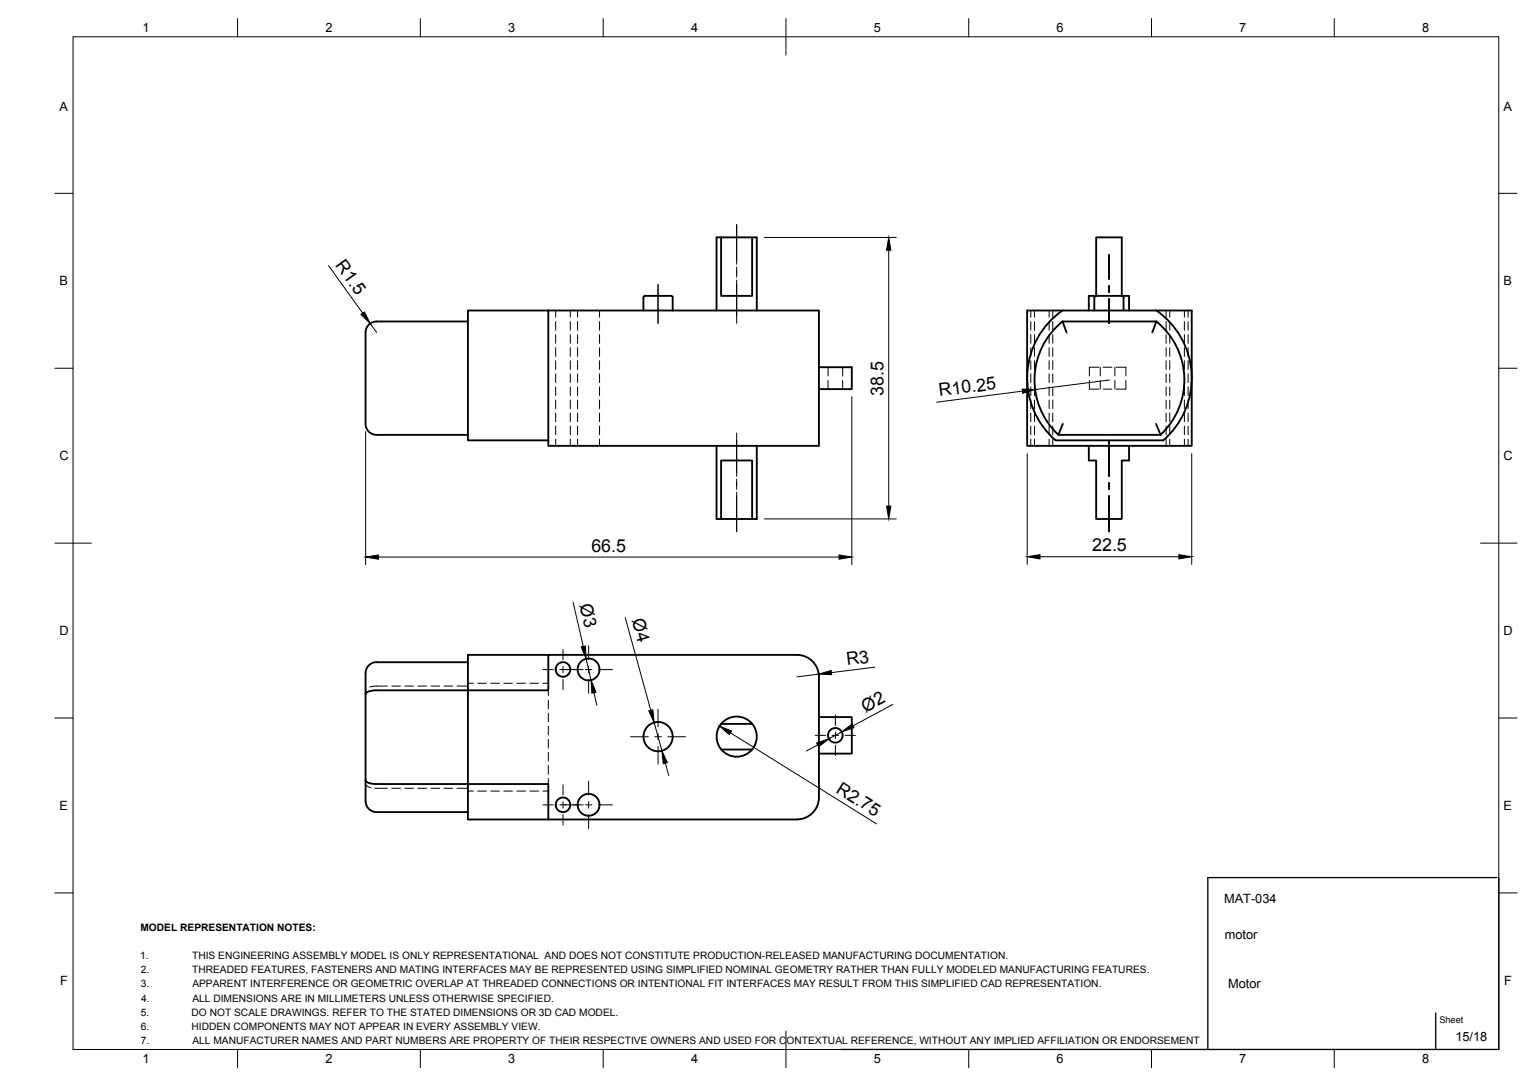
ISO-10303-21;
HEADER;
/* Generated by software containing ST-Developer
 * from STEP Tools, Inc. (www.steptools.com) 
 */

FILE_DESCRIPTION(
/* description */ ('STEP AP214'),
/* implementation_level */ '2;1');

FILE_NAME(
/* name */ 'Motor.step',
/* time_stamp */ '2026-11-14T09:24:36-08:00',
/* author */ (''),
/* organization */ (''),
/* preprocessor_version */ 'ST-DEVELOPER v20.2',
/* originating_system */ 'Autodesk Translation Framework v15.17.0.0',
/* authorisation */ '');

FILE_SCHEMA (('AUTOMOTIVE_DESIGN { 1 0 10303 214 3 1 1 }'));
ENDSEC;

DATA;
#10=MECHANICAL_DESIGN_GEOMETRIC_PRESENTATION_REPRESENTATION('',(#210),#18867);
#142=B_SPLINE_CURVE_WITH_KNOTS('',3,(#16841,#16842,#16843,#16844,#16845,
#16846,#16847,#16848,#16849,#16850,#16851,#16852,#16853,#16854),
 .UNSPECIFIED.,.F.,.F.,(4,2,2,2,2,2,4),(0.245799129465821,0.300704982929502,
0.357513955396153,0.418543136612542,0.45489286030411,0.491598258931638,
0.492200531214483),.UNSPECIFIED.);
#143=B_SPLINE_CURVE_WITH_KNOTS('',3,(#16857,#16858,#16859,#16860,#16861,
#16862,#16863,#16864,#16865,#16866,#16867,#16868,#16869,#16870),
 .UNSPECIFIED.,.F.,.F.,(4,2,2,2,2,2,4),(-0.243764588636152,-0.188160877929009,
-0.130985417478992,-0.0703706382818566,-0.0353193180725583,0.,0.000595335954832901),
 .UNSPECIFIED.);
#144=B_SPLINE_CURVE_WITH_KNOTS('',3,(#17002,#17003,#17004,#17005,#17006,
#17007,#17008,#17009,#17010,#17011,#17012,#17013,#17014,#17015),
 .UNSPECIFIED.,.F.,.F.,(4,2,2,2,2,2,4),(-0.000602272282836634,0.,0.0367053986270638,
0.0730551223181225,0.134084303533662,0.190893275999521,0.245799129462431),
 .UNSPECIFIED.);
#145=B_SPLINE_CURVE_WITH_KNOTS('',3,(#17017,#17018,#17019,#17020,#17021,
#17022,#17023,#17024,#17025,#17026,#17027,#17028,#17029,#17030),
 .UNSPECIFIED.,.F.,.F.,(4,2,2,2,2,2,4),(-0.488124513225642,-0.487529177270534,
-0.452209859198347,-0.417158538989302,-0.356543759792373,-0.299368299342555,
-0.243764588635598),.UNSPECIFIED.);
#154=TOROIDAL_SURFACE('',#11579,1.8,0.2);
#155=TOROIDAL_SURFACE('',#11608,8.75000000000038,1.5);
#156=TOROIDAL_SURFACE('',#11653,8.75000000000038,1.5);
#178=SHAPE_REPRESENTATION_RELATIONSHIP('SRR','None',#18942,#194);
#194=ADVANCED_BREP_SHAPE_REPRESENTATION('',(#234),#18858);
#210=STYLED_ITEM('',(#19026),#234);
#234=MANIFOLD_SOLID_BREP('Body1',#10965);
#327=FACE_BOUND('',#1639,.T.);
#328=FACE_BOUND('',#1640,.T.);
#329=FACE_BOUND('',#1641,.T.);
#330=FACE_BOUND('',#1642,.T.);
#331=FACE_BOUND('',#1643,.T.);
#332=FACE_BOUND('',#1644,.T.);
#333=FACE_BOUND('',#1646,.T.);
#334=FACE_BOUND('',#1649,.T.);
#335=FACE_BOUND('',#1659,.T.);
#336=FACE_BOUND('',#1660,.T.);
#337=FACE_BOUND('',#1661,.T.);
#338=FACE_BOUND('',#1662,.T.);
#339=FACE_BOUND('',#1663,.T.);
#340=FACE_BOUND('',#1682,.T.);
#341=FACE_BOUND('',#1685,.T.);
#523=PLANE('',#11625);
#524=PLANE('',#11628);
#525=PLANE('',#11629);
#526=PLANE('',#11630);
#527=PLANE('',#11636);
#528=PLANE('',#11637);
#529=PLANE('',#11638);
#530=PLANE('',#11639);
#531=PLANE('',#11644);
#532=PLANE('',#11645);
#533=PLANE('',#11646);
#534=PLANE('',#11648);
#535=PLANE('',#11649);
#536=PLANE('',#11650);
#537=PLANE('',#11655);
#538=PLANE('',#11656);
#539=PLANE('',#11657);
#540=PLANE('',#11658);
#541=PLANE('',#11659);
#542=PLANE('',#11660);
#543=PLANE('',#11661);
#544=PLANE('',#11662);
#545=PLANE('',#11663);
#546=PLANE('',#11664);
#547=PLANE('',#11665);
#548=PLANE('',#11666);
#549=PLANE('',#11667);
#550=PLANE('',#11668);
#551=PLANE('',#11669);
#954=FACE_OUTER_BOUND('',#1626,.T.);
#955=FACE_OUTER_BOUND('',#1627,.T.);
#956=FACE_OUTER_BOUND('',#1628,.T.);
#957=FACE_OUTER_BOUND('',#1629,.T.);
#958=FACE_OUTER_BOUND('',#1630,.T.);
#959=FACE_OUTER_BOUND('',#1631,.T.);
#960=FACE_OUTER_BOUND('',#1632,.T.);
#961=FACE_OUTER_BOUND('',#1633,.T.);
#962=FACE_OUTER_BOUND('',#1634,.T.);
#963=FACE_OUTER_BOUND('',#1635,.T.);
#964=FACE_OUTER_BOUND('',#1636,.T.);
#965=FACE_OUTER_BOUND('',#1637,.T.);
#966=FACE_OUTER_BOUND('',#1638,.T.);
#967=FACE_OUTER_BOUND('',#1645,.T.);
#968=FACE_OUTER_BOUND('',#1647,.T.);
#969=FACE_OUTER_BOUND('',#1648,.T.);
#970=FACE_OUTER_BOUND('',#1650,.T.);
#971=FACE_OUTER_BOUND('',#1651,.T.);
#972=FACE_OUTER_BOUND('',#1652,.T.);
#973=FACE_OUTER_BOUND('',#1653,.T.);
#974=FACE_OUTER_BOUND('',#1654,.T.);
#975=FACE_OUTER_BOUND('',#1655,.T.);
#976=FACE_OUTER_BOUND('',#1656,.T.);
#977=FACE_OUTER_BOUND('',#1657,.T.);
#978=FACE_OUTER_BOUND('',#1658,.T.);
#979=FACE_OUTER_BOUND('',#1664,.T.);
#980=FACE_OUTER_BOUND('',#1665,.T.);
#981=FACE_OUTER_BOUND('',#1666,.T.);
#982=FACE_OUTER_BOUND('',#1667,.T.);
#983=FACE_OUTER_BOUND('',#1668,.T.);
#984=FACE_OUTER_BOUND('',#1669,.T.);
#985=FACE_OUTER_BOUND('',#1670,.T.);
#986=FACE_OUTER_BOUND('',#1671,.T.);
#987=FACE_OUTER_BOUND('',#1672,.T.);
#988=FACE_OUTER_BOUND('',#1673,.T.);
#989=FACE_OUTER_BOUND('',#1674,.T.);
#990=FACE_OUTER_BOUND('',#1675,.T.);
#991=FACE_OUTER_BOUND('',#1676,.T.);
#992=FACE_OUTER_BOUND('',#1677,.T.);
#993=FACE_OUTER_BOUND('',#1678,.T.);
#994=FACE_OUTER_BOUND('',#1679,.T.);
#995=FACE_OUTER_BOUND('',#1680,.T.);
#996=FACE_OUTER_BOUND('',#1681,.T.);
#997=FACE_OUTER_BOUND('',#1683,.T.);
#998=FACE_OUTER_BOUND('',#1684,.T.);
#999=FACE_OUTER_BOUND('',#1686,.T.);
#1000=FACE_OUTER_BOUND('',#1687,.T.);
#1001=FACE_OUTER_BOUND('',#1688,.T.);
#1626=EDGE_LOOP('',(#8226,#8227,#8228,#8229,#8230));
#1627=EDGE_LOOP('',(#8231,#8232,#8233,#8234,#8235));
#1628=EDGE_LOOP('',(#8236,#8237,#8238,#8239));
#1629=EDGE_LOOP('',(#8240,#8241,#8242,#8243));
#1630=EDGE_LOOP('',(#8244,#8245,#8246,#8247));
#1631=EDGE_LOOP('',(#8248,#8249,#8250,#8251));
#1632=EDGE_LOOP('',(#8252,#8253,#8254,#8255));
#1633=EDGE_LOOP('',(#8256,#8257,#8258,#8259,#8260,#8261,#8262,#8263,#8264,
#8265,#8266,#8267));
#1634=EDGE_LOOP('',(#8268,#8269,#8270,#8271));
#1635=EDGE_LOOP('',(#8272,#8273,#8274,#8275));
#1636=EDGE_LOOP('',(#8276,#8277,#8278,#8279,#8280));
#1637=EDGE_LOOP('',(#8281,#8282,#8283,#8284,#8285,#8286,#8287,#8288,#8289,
#8290,#8291,#8292));
#1638=EDGE_LOOP('',(#8293,#8294,#8295,#8296,#8297,#8298,#8299,#8300,#8301,
#8302));
#1639=EDGE_LOOP('',(#8303));
#1640=EDGE_LOOP('',(#8304));
#1641=EDGE_LOOP('',(#8305));
#1642=EDGE_LOOP('',(#8306));
#1643=EDGE_LOOP('',(#8307));
#1644=EDGE_LOOP('',(#8308));
#1645=EDGE_LOOP('',(#8309,#8310,#8311,#8312));
#1646=EDGE_LOOP('',(#8313,#8314,#8315,#8316));
#1647=EDGE_LOOP('',(#8317,#8318,#8319,#8320,#8321));
#1648=EDGE_LOOP('',(#8322,#8323,#8324,#8325));
#1649=EDGE_LOOP('',(#8326,#8327,#8328,#8329));
#1650=EDGE_LOOP('',(#8330,#8331,#8332,#8333,#8334));
#1651=EDGE_LOOP('',(#8335,#8336,#8337));
#1652=EDGE_LOOP('',(#8338,#8339,#8340,#8341,#8342,#8343));
#1653=EDGE_LOOP('',(#8344,#8345,#8346));
#1654=EDGE_LOOP('',(#8347,#8348,#8349,#8350,#8351));
#1655=EDGE_LOOP('',(#8352,#8353,#8354,#8355));
#1656=EDGE_LOOP('',(#8356,#8357,#8358,#8359));
#1657=EDGE_LOOP('',(#8360,#8361,#8362,#8363,#8364));
#1658=EDGE_LOOP('',(#8365,#8366,#8367,#8368,#8369,#8370));
#1659=EDGE_LOOP('',(#8371));
#1660=EDGE_LOOP('',(#8372));
#1661=EDGE_LOOP('',(#8373));
#1662=EDGE_LOOP('',(#8374));
#1663=EDGE_LOOP('',(#8375));
#1664=EDGE_LOOP('',(#8376,#8377,#8378,#8379));
#1665=EDGE_LOOP('',(#8380,#8381,#8382,#8383));
#1666=EDGE_LOOP('',(#8384,#8385,#8386,#8387));
#1667=EDGE_LOOP('',(#8388,#8389,#8390,#8391));
#1668=EDGE_LOOP('',(#8392,#8393,#8394,#8395));
#1669=EDGE_LOOP('',(#8396,#8397,#8398,#8399));
#1670=EDGE_LOOP('',(#8400,#8401,#8402,#8403));
#1671=EDGE_LOOP('',(#8404,#8405,#8406,#8407));
#1672=EDGE_LOOP('',(#8408,#8409,#8410,#8411,#8412));
#1673=EDGE_LOOP('',(#8413,#8414));
#1674=EDGE_LOOP('',(#8415,#8416,#8417,#8418));
#1675=EDGE_LOOP('',(#8419,#8420));
#1676=EDGE_LOOP('',(#8421,#8422,#8423,#8424));
#1677=EDGE_LOOP('',(#8425,#8426,#8427,#8428));
#1678=EDGE_LOOP('',(#8429,#8430));
#1679=EDGE_LOOP('',(#8431,#8432,#8433,#8434));
#1680=EDGE_LOOP('',(#8435,#8436));
#1681=EDGE_LOOP('',(#8437,#8438,#8439,#8440));
#1682=EDGE_LOOP('',(#8441));
#1683=EDGE_LOOP('',(#8442,#8443,#8444,#8445));
#1684=EDGE_LOOP('',(#8446,#8447,#8448,#8449));
#1685=EDGE_LOOP('',(#8450));
#1686=EDGE_LOOP('',(#8451,#8452,#8453,#8454));
#1687=EDGE_LOOP('',(#8455,#8456,#8457,#8458));
#1688=EDGE_LOOP('',(#8459));
#2424=LINE('',#16783,#3438);
#2425=LINE('',#16788,#3439);
#2426=LINE('',#16794,#3440);
#2427=LINE('',#16800,#3441);
#2428=LINE('',#16806,#3442);
#2429=LINE('',#16812,#3443);
#2430=LINE('',#16818,#3444);
#2431=LINE('',#16822,#3445);
#2432=LINE('',#16826,#3446);
#2433=LINE('',#16830,#3447);
#2434=LINE('',#16834,#3448);
#2435=LINE('',#16876,#3449);
#2436=LINE('',#16879,#3450);
#2437=LINE('',#16885,#3451);
#2438=LINE('',#16890,#3452);
#2439=LINE('',#16895,#3453);
#2440=LINE('',#16899,#3454);
#2441=LINE('',#16903,#3455);
#2442=LINE('',#16907,#3456);
#2443=LINE('',#16911,#3457);
#2444=LINE('',#16915,#3458);
#2445=LINE('',#16917,#3459);
#2446=LINE('',#16921,#3460);
#2447=LINE('',#16925,#3461);
#2448=LINE('',#16927,#3462);
#2449=LINE('',#16929,#3463);
#2450=LINE('',#16930,#3464);
#2451=LINE('',#16934,#3465);
#2452=LINE('',#16935,#3466);
#2453=LINE('',#16936,#3467);
#2454=LINE('',#16939,#3468);
#2455=LINE('',#16941,#3469);
#2456=LINE('',#16943,#3470);
#2457=LINE('',#16944,#3471);
#2458=LINE('',#16946,#3472);
#2459=LINE('',#16947,#3473);
#2460=LINE('',#16951,#3474);
#2461=LINE('',#16953,#3475);
#2462=LINE('',#16956,#3476);
#2463=LINE('',#16962,#3477);
#2464=LINE('',#16964,#3478);
#2465=LINE('',#16967,#3479);
#2466=LINE('',#16969,#3480);
#2467=LINE('',#16970,#3481);
#2468=LINE('',#16971,#3482);
#2469=LINE('',#16973,#3483);
#2470=LINE('',#16976,#3484);
#2471=LINE('',#16977,#3485);
#2472=LINE('',#16983,#3486);
#2473=LINE('',#16985,#3487);
#2474=LINE('',#16989,#3488);
#2475=LINE('',#16990,#3489);
#2476=LINE('',#16992,#3490);
#2477=LINE('',#16994,#3491);
#2478=LINE('',#16999,#3492);
#2479=LINE('',#17000,#3493);
#2480=LINE('',#17033,#3494);
#2481=LINE('',#17034,#3495);
#2482=LINE('',#17036,#3496);
#2483=LINE('',#17039,#3497);
#2484=LINE('',#17042,#3498);
#2485=LINE('',#17045,#3499);
#2486=LINE('',#17049,#3500);
#2487=LINE('',#17051,#3501);
#2488=LINE('',#17052,#3502);
#2489=LINE('',#17055,#3503);
#2490=LINE('',#17056,#3504);
#2491=LINE('',#17059,#3505);
#2492=LINE('',#17060,#3506);
#2493=LINE('',#17062,#3507);
#3438=VECTOR('',#13534,2.);
#3439=VECTOR('',#13539,1.);
#3440=VECTOR('',#13546,1.);
#3441=VECTOR('',#13553,1.5);
#3442=VECTOR('',#13560,1.5);
#3443=VECTOR('',#13567,1.);
#3444=VECTOR('',#13574,2.75);
#3445=VECTOR('',#13577,1000.);
#3446=VECTOR('',#13580,1000.);
#3447=VECTOR('',#13583,1000.);
#3448=VECTOR('',#13586,1000.);
#3449=VECTOR('',#13599,1000.);
#3450=VECTOR('',#13602,1000.);
#3451=VECTOR('',#13607,1000.);
#3452=VECTOR('',#13612,1000.);
#3453=VECTOR('',#13617,2.75);
#3454=VECTOR('',#13620,1000.);
#3455=VECTOR('',#13623,1000.);
#3456=VECTOR('',#13626,1000.);
#3457=VECTOR('',#13629,1000.);
#3458=VECTOR('',#13634,1000.);
#3459=VECTOR('',#13635,1000.);
#3460=VECTOR('',#13638,1000.);
#3461=VECTOR('',#13641,1000.);
#3462=VECTOR('',#13642,1000.);
#3463=VECTOR('',#13643,1000.);
#3464=VECTOR('',#13644,1000.);
#3465=VECTOR('',#13647,1000.);
#3466=VECTOR('',#13648,1000.);
#3467=VECTOR('',#13649,1000.);
#3468=VECTOR('',#13650,1000.);
#3469=VECTOR('',#13651,1000.);
#3470=VECTOR('',#13652,1000.);
#3471=VECTOR('',#13653,1000.);
#3472=VECTOR('',#13656,1000.);
#3473=VECTOR('',#13657,1000.);
#3474=VECTOR('',#13662,1000.);
#3475=VECTOR('',#13663,1000.);
#3476=VECTOR('',#13666,1000.);
#3477=VECTOR('',#13673,1000.);
#3478=VECTOR('',#13676,1000.);
#3479=VECTOR('',#13679,1000.);
#3480=VECTOR('',#13680,1000.);
#3481=VECTOR('',#13681,1000.);
#3482=VECTOR('',#13682,1000.);
#3483=VECTOR('',#13685,1000.);
#3484=VECTOR('',#13688,1000.);
#3485=VECTOR('',#13689,1000.);
#3486=VECTOR('',#13698,1000.);
#3487=VECTOR('',#13701,1000.);
#3488=VECTOR('',#13708,1000.);
#3489=VECTOR('',#13709,1000.);
#3490=VECTOR('',#13712,1000.);
#3491=VECTOR('',#13715,1000.);
#3492=VECTOR('',#13720,1000.);
#3493=VECTOR('',#13721,1000.);
#3494=VECTOR('',#13730,1000.);
#3495=VECTOR('',#13731,1000.);
#3496=VECTOR('',#13734,1000.);
#3497=VECTOR('',#13739,1000.);
#3498=VECTOR('',#13744,1000.);
#3499=VECTOR('',#13749,1000.);
#3500=VECTOR('',#13754,1000.);
#3501=VECTOR('',#13755,1000.);
#3502=VECTOR('',#13756,1000.);
#3503=VECTOR('',#13759,1000.);
#3504=VECTOR('',#13760,1000.);
#3505=VECTOR('',#13763,1000.);
#3506=VECTOR('',#13764,1000.);
#3507=VECTOR('',#13767,1000.);
#4253=CIRCLE('',#11580,1.8);
#4254=CIRCLE('',#11581,0.2);
#4255=CIRCLE('',#11582,2.);
#4256=CIRCLE('',#11583,2.);
#4257=CIRCLE('',#11585,2.);
#4258=CIRCLE('',#11587,1.);
#4259=CIRCLE('',#11588,1.);
#4260=CIRCLE('',#11590,1.);
#4261=CIRCLE('',#11591,1.);
#4262=CIRCLE('',#11593,1.5);
#4263=CIRCLE('',#11594,1.5);
#4264=CIRCLE('',#11596,1.5);
#4265=CIRCLE('',#11597,1.5);
#4266=CIRCLE('',#11599,1.);
#4267=CIRCLE('',#11600,1.);
#4268=CIRCLE('',#11602,2.75);
#4269=CIRCLE('',#11603,2.75);
#4270=CIRCLE('',#11604,2.75);
#4271=CIRCLE('',#11605,2.75);
#4272=CIRCLE('',#11606,2.75);
#4273=CIRCLE('',#11607,2.75);
#4274=CIRCLE('',#11609,10.2500000000004);
#4275=CIRCLE('',#11610,8.75000000000038);
#4276=CIRCLE('',#11612,10.2500000000004);
#4277=CIRCLE('',#11613,10.2500000000004);
#4278=CIRCLE('',#11615,11.25);
#4279=CIRCLE('',#11616,11.25);
#4280=CIRCLE('',#11617,11.25);
#4281=CIRCLE('',#11619,2.75);
#4282=CIRCLE('',#11620,2.75);
#4283=CIRCLE('',#11621,2.75);
#4284=CIRCLE('',#11622,2.75);
#4285=CIRCLE('',#11623,2.75);
#4286=CIRCLE('',#11624,2.75);
#4287=CIRCLE('',#11626,3.);
#4288=CIRCLE('',#11627,3.);
#4289=CIRCLE('',#11631,11.25);
#4290=CIRCLE('',#11632,10.2500000000004);
#4291=CIRCLE('',#11634,11.25);
#4292=CIRCLE('',#11635,11.25);
#4293=CIRCLE('',#11641,3.);
#4294=CIRCLE('',#11643,3.);
#4295=CIRCLE('',#11651,8.75000000000038);
#4944=VERTEX_POINT('',#16773);
#4945=VERTEX_POINT('',#16775);
#4946=VERTEX_POINT('',#16777);
#4947=VERTEX_POINT('',#16781);
#4948=VERTEX_POINT('',#16785);
#4949=VERTEX_POINT('',#16787);
#4950=VERTEX_POINT('',#16791);
#4951=VERTEX_POINT('',#16793);
#4952=VERTEX_POINT('',#16797);
#4953=VERTEX_POINT('',#16799);
#4954=VERTEX_POINT('',#16803);
#4955=VERTEX_POINT('',#16805);
#4956=VERTEX_POINT('',#16809);
#4957=VERTEX_POINT('',#16811);
#4958=VERTEX_POINT('',#16815);
#4959=VERTEX_POINT('',#16817);
#4960=VERTEX_POINT('',#16819);
#4961=VERTEX_POINT('',#16821);
#4962=VERTEX_POINT('',#16823);
#4963=VERTEX_POINT('',#16825);
#4964=VERTEX_POINT('',#16827);
#4965=VERTEX_POINT('',#16829);
#4966=VERTEX_POINT('',#16831);
#4967=VERTEX_POINT('',#16833);
#4968=VERTEX_POINT('',#16837);
#4969=VERTEX_POINT('',#16838);
#4970=VERTEX_POINT('',#16840);
#4971=VERTEX_POINT('',#16855);
#4972=VERTEX_POINT('',#16872);
#4973=VERTEX_POINT('',#16873);
#4974=VERTEX_POINT('',#16875);
#4975=VERTEX_POINT('',#16877);
#4976=VERTEX_POINT('',#16881);
#4977=VERTEX_POINT('',#16882);
#4978=VERTEX_POINT('',#16884);
#4979=VERTEX_POINT('',#16886);
#4980=VERTEX_POINT('',#16888);
#4981=VERTEX_POINT('',#16892);
#4982=VERTEX_POINT('',#16894);
#4983=VERTEX_POINT('',#16896);
#4984=VERTEX_POINT('',#16898);
#4985=VERTEX_POINT('',#16900);
#4986=VERTEX_POINT('',#16902);
#4987=VERTEX_POINT('',#16904);
#4988=VERTEX_POINT('',#16906);
#4989=VERTEX_POINT('',#16908);
#4990=VERTEX_POINT('',#16910);
#4991=VERTEX_POINT('',#16914);
#4992=VERTEX_POINT('',#16916);
#4993=VERTEX_POINT('',#16918);
#4994=VERTEX_POINT('',#16920);
#4995=VERTEX_POINT('',#16922);
#4996=VERTEX_POINT('',#16924);
#4997=VERTEX_POINT('',#16926);
#4998=VERTEX_POINT('',#16928);
#4999=VERTEX_POINT('',#16932);
#5000=VERTEX_POINT('',#16933);
#5001=VERTEX_POINT('',#16937);
#5002=VERTEX_POINT('',#16938);
#5003=VERTEX_POINT('',#16940);
#5004=VERTEX_POINT('',#16942);
#5005=VERTEX_POINT('',#16949);
#5006=VERTEX_POINT('',#16952);
#5007=VERTEX_POINT('',#16954);
#5008=VERTEX_POINT('',#16958);
#5009=VERTEX_POINT('',#16960);
#5010=VERTEX_POINT('',#16966);
#5011=VERTEX_POINT('',#16968);
#5012=VERTEX_POINT('',#16975);
#5013=VERTEX_POINT('',#16981);
#5014=VERTEX_POINT('',#16996);
#5015=VERTEX_POINT('',#16997);
#5016=VERTEX_POINT('',#17048);
#5017=VERTEX_POINT('',#17050);
#5018=VERTEX_POINT('',#17054);
#5019=VERTEX_POINT('',#17058);
#6146=EDGE_CURVE('',#4944,#4944,#4253,.T.);
#6147=EDGE_CURVE('',#4944,#4945,#4254,.T.);
#6148=EDGE_CURVE('',#4946,#4945,#4255,.T.);
#6149=EDGE_CURVE('',#4945,#4946,#4256,.T.);
#6150=EDGE_CURVE('',#4947,#4947,#4257,.T.);
#6151=EDGE_CURVE('',#4947,#4946,#2424,.T.);
#6152=EDGE_CURVE('',#4948,#4948,#4258,.T.);
#6153=EDGE_CURVE('',#4948,#4949,#2425,.T.);
#6154=EDGE_CURVE('',#4949,#4949,#4259,.T.);
#6155=EDGE_CURVE('',#4950,#4950,#4260,.T.);
#6156=EDGE_CURVE('',#4950,#4951,#2426,.T.);
#6157=EDGE_CURVE('',#4951,#4951,#4261,.T.);
#6158=EDGE_CURVE('',#4952,#4952,#4262,.T.);
#6159=EDGE_CURVE('',#4952,#4953,#2427,.T.);
#6160=EDGE_CURVE('',#4953,#4953,#4263,.T.);
#6161=EDGE_CURVE('',#4954,#4954,#4264,.T.);
#6162=EDGE_CURVE('',#4954,#4955,#2428,.T.);
#6163=EDGE_CURVE('',#4955,#4955,#4265,.T.);
#6164=EDGE_CURVE('',#4956,#4956,#4266,.T.);
#6165=EDGE_CURVE('',#4956,#4957,#2429,.T.);
#6166=EDGE_CURVE('',#4957,#4957,#4267,.T.);
#6167=EDGE_CURVE('',#4958,#4958,#4268,.T.);
#6168=EDGE_CURVE('',#4958,#4959,#2430,.T.);
#6169=EDGE_CURVE('',#4960,#4959,#4269,.T.);
#6170=EDGE_CURVE('',#4960,#4961,#2431,.T.);
#6171=EDGE_CURVE('',#4962,#4961,#4270,.T.);
#6172=EDGE_CURVE('',#4962,#4963,#2432,.T.);
#6173=EDGE_CURVE('',#4964,#4963,#4271,.T.);
#6174=EDGE_CURVE('',#4964,#4965,#2433,.T.);
#6175=EDGE_CURVE('',#4966,#4965,#4272,.T.);
#6176=EDGE_CURVE('',#4966,#4967,#2434,.T.);
#6177=EDGE_CURVE('',#4959,#4967,#4273,.T.);
#6178=EDGE_CURVE('',#4968,#4969,#4274,.T.);
#6179=EDGE_CURVE('',#4968,#4970,#142,.T.);
#6180=EDGE_CURVE('',#4971,#4970,#4275,.T.);
#6181=EDGE_CURVE('',#4969,#4971,#143,.T.);
#6182=EDGE_CURVE('',#4972,#4973,#4276,.T.);
#6183=EDGE_CURVE('',#4973,#4974,#2435,.T.);
#6184=EDGE_CURVE('',#4974,#4975,#4277,.T.);
#6185=EDGE_CURVE('',#4972,#4975,#2436,.T.);
#6186=EDGE_CURVE('',#4976,#4977,#4278,.T.);
#6187=EDGE_CURVE('',#4976,#4978,#2437,.T.);
#6188=EDGE_CURVE('',#4978,#4979,#4279,.T.);
#6189=EDGE_CURVE('',#4979,#4980,#4280,.T.);
#6190=EDGE_CURVE('',#4980,#4977,#2438,.T.);
#6191=EDGE_CURVE('',#4981,#4981,#4281,.T.);
#6192=EDGE_CURVE('',#4981,#4982,#2439,.T.);
#6193=EDGE_CURVE('',#4982,#4983,#4282,.T.);
#6194=EDGE_CURVE('',#4983,#4984,#2440,.T.);
#6195=EDGE_CURVE('',#4984,#4985,#4283,.T.);
#6196=EDGE_CURVE('',#4985,#4986,#2441,.T.);
#6197=EDGE_CURVE('',#4986,#4987,#4284,.T.);
#6198=EDGE_CURVE('',#4987,#4988,#2442,.T.);
#6199=EDGE_CURVE('',#4988,#4989,#4285,.T.);
#6200=EDGE_CURVE('',#4989,#4990,#2443,.T.);
#6201=EDGE_CURVE('',#4990,#4982,#4286,.T.);
#6202=EDGE_CURVE('',#4991,#4980,#2444,.T.);
#6203=EDGE_CURVE('',#4992,#4991,#2445,.T.);
#6204=EDGE_CURVE('',#4993,#4992,#4287,.T.);
#6205=EDGE_CURVE('',#4994,#4993,#2446,.T.);
#6206=EDGE_CURVE('',#4995,#4994,#4288,.T.);
#6207=EDGE_CURVE('',#4996,#4995,#2447,.T.);
#6208=EDGE_CURVE('',#4997,#4996,#2448,.T.);
#6209=EDGE_CURVE('',#4998,#4997,#2449,.T.);
#6210=EDGE_CURVE('',#4998,#4977,#2450,.T.);
#6211=EDGE_CURVE('',#4999,#5000,#2451,.T.);
#6212=EDGE_CURVE('',#4994,#4999,#2452,.T.);
#6213=EDGE_CURVE('',#4993,#5000,#2453,.T.);
#6214=EDGE_CURVE('',#5001,#5002,#2454,.T.);
#6215=EDGE_CURVE('',#5003,#5001,#2455,.T.);
#6216=EDGE_CURVE('',#5004,#5003,#2456,.T.);
#6217=EDGE_CURVE('',#5002,#5004,#2457,.T.);
#6218=EDGE_CURVE('',#4986,#4983,#2458,.T.);
#6219=EDGE_CURVE('',#4990,#4987,#2459,.T.);
#6220=EDGE_CURVE('',#4998,#5005,#4289,.T.);
#6221=EDGE_CURVE('',#4976,#5005,#2460,.T.);
#6222=EDGE_CURVE('',#5006,#4974,#2461,.T.);
#6223=EDGE_CURVE('',#5007,#5006,#4290,.T.);
#6224=EDGE_CURVE('',#4975,#5007,#2462,.T.);
#6225=EDGE_CURVE('',#4997,#5008,#4291,.T.);
#6226=EDGE_CURVE('',#5008,#5009,#4292,.T.);
#6227=EDGE_CURVE('',#5009,#5005,#2463,.T.);
#6228=EDGE_CURVE('',#4991,#4979,#2464,.T.);
#6229=EDGE_CURVE('',#5008,#5010,#2465,.T.);
#6230=EDGE_CURVE('',#5011,#5010,#2466,.T.);
#6231=EDGE_CURVE('',#4979,#5011,#2467,.T.);
#6232=EDGE_CURVE('',#4978,#5009,#2468,.T.);
#6233=EDGE_CURVE('',#4996,#5008,#2469,.T.);
#6234=EDGE_CURVE('',#5012,#5011,#2470,.T.);
#6235=EDGE_CURVE('',#4992,#5012,#2471,.T.);
#6236=EDGE_CURVE('',#5000,#5012,#4293,.T.);
#6237=EDGE_CURVE('',#5013,#4999,#4294,.T.);
#6238=EDGE_CURVE('',#4995,#5013,#2472,.T.);
#6239=EDGE_CURVE('',#5010,#5013,#2473,.T.);
#6240=EDGE_CURVE('',#4968,#5006,#2474,.T.);
#6241=EDGE_CURVE('',#4969,#5007,#2475,.T.);
#6242=EDGE_CURVE('',#4973,#4968,#2476,.T.);
#6243=EDGE_CURVE('',#4969,#4972,#2477,.T.);
#6244=EDGE_CURVE('',#5014,#5015,#4295,.T.);
#6245=EDGE_CURVE('',#5015,#4971,#2478,.T.);
#6246=EDGE_CURVE('',#4970,#5014,#2479,.T.);
#6247=EDGE_CURVE('',#5014,#4973,#144,.T.);
#6248=EDGE_CURVE('',#5015,#4972,#145,.T.);
#6249=EDGE_CURVE('',#4960,#4963,#2480,.T.);
#6250=EDGE_CURVE('',#4964,#4967,#2481,.T.);
#6251=EDGE_CURVE('',#4965,#4966,#2482,.T.);
#6252=EDGE_CURVE('',#4961,#4962,#2483,.T.);
#6253=EDGE_CURVE('',#4989,#4988,#2484,.T.);
#6254=EDGE_CURVE('',#4985,#4984,#2485,.T.);
#6255=EDGE_CURVE('',#5016,#5001,#2486,.T.);
#6256=EDGE_CURVE('',#5017,#5016,#2487,.T.);
#6257=EDGE_CURVE('',#5017,#5003,#2488,.T.);
#6258=EDGE_CURVE('',#5018,#5002,#2489,.T.);
#6259=EDGE_CURVE('',#5016,#5018,#2490,.T.);
#6260=EDGE_CURVE('',#5019,#5004,#2491,.T.);
#6261=EDGE_CURVE('',#5018,#5019,#2492,.T.);
#6262=EDGE_CURVE('',#5019,#5017,#2493,.T.);
#8226=ORIENTED_EDGE('',*,*,#6146,.F.);
#8227=ORIENTED_EDGE('',*,*,#6147,.T.);
#8228=ORIENTED_EDGE('',*,*,#6148,.F.);
#8229=ORIENTED_EDGE('',*,*,#6149,.F.);
#8230=ORIENTED_EDGE('',*,*,#6147,.F.);
#8231=ORIENTED_EDGE('',*,*,#6150,.T.);
#8232=ORIENTED_EDGE('',*,*,#6151,.T.);
#8233=ORIENTED_EDGE('',*,*,#6148,.T.);
#8234=ORIENTED_EDGE('',*,*,#6149,.T.);
#8235=ORIENTED_EDGE('',*,*,#6151,.F.);
#8236=ORIENTED_EDGE('',*,*,#6152,.F.);
#8237=ORIENTED_EDGE('',*,*,#6153,.T.);
#8238=ORIENTED_EDGE('',*,*,#6154,.T.);
#8239=ORIENTED_EDGE('',*,*,#6153,.F.);
#8240=ORIENTED_EDGE('',*,*,#6155,.F.);
#8241=ORIENTED_EDGE('',*,*,#6156,.T.);
#8242=ORIENTED_EDGE('',*,*,#6157,.T.);
#8243=ORIENTED_EDGE('',*,*,#6156,.F.);
#8244=ORIENTED_EDGE('',*,*,#6158,.F.);
#8245=ORIENTED_EDGE('',*,*,#6159,.T.);
#8246=ORIENTED_EDGE('',*,*,#6160,.T.);
#8247=ORIENTED_EDGE('',*,*,#6159,.F.);
#8248=ORIENTED_EDGE('',*,*,#6161,.F.);
#8249=ORIENTED_EDGE('',*,*,#6162,.T.);
#8250=ORIENTED_EDGE('',*,*,#6163,.T.);
#8251=ORIENTED_EDGE('',*,*,#6162,.F.);
#8252=ORIENTED_EDGE('',*,*,#6164,.T.);
#8253=ORIENTED_EDGE('',*,*,#6165,.T.);
#8254=ORIENTED_EDGE('',*,*,#6166,.T.);
#8255=ORIENTED_EDGE('',*,*,#6165,.F.);
#8256=ORIENTED_EDGE('',*,*,#6167,.T.);
#8257=ORIENTED_EDGE('',*,*,#6168,.T.);
#8258=ORIENTED_EDGE('',*,*,#6169,.F.);
#8259=ORIENTED_EDGE('',*,*,#6170,.T.);
#8260=ORIENTED_EDGE('',*,*,#6171,.F.);
#8261=ORIENTED_EDGE('',*,*,#6172,.T.);
#8262=ORIENTED_EDGE('',*,*,#6173,.F.);
#8263=ORIENTED_EDGE('',*,*,#6174,.T.);
#8264=ORIENTED_EDGE('',*,*,#6175,.F.);
#8265=ORIENTED_EDGE('',*,*,#6176,.T.);
#8266=ORIENTED_EDGE('',*,*,#6177,.F.);
#8267=ORIENTED_EDGE('',*,*,#6168,.F.);
#8268=ORIENTED_EDGE('',*,*,#6178,.F.);
#8269=ORIENTED_EDGE('',*,*,#6179,.T.);
#8270=ORIENTED_EDGE('',*,*,#6180,.F.);
#8271=ORIENTED_EDGE('',*,*,#6181,.F.);
#8272=ORIENTED_EDGE('',*,*,#6182,.T.);
#8273=ORIENTED_EDGE('',*,*,#6183,.T.);
#8274=ORIENTED_EDGE('',*,*,#6184,.T.);
#8275=ORIENTED_EDGE('',*,*,#6185,.F.);
#8276=ORIENTED_EDGE('',*,*,#6186,.F.);
#8277=ORIENTED_EDGE('',*,*,#6187,.T.);
#8278=ORIENTED_EDGE('',*,*,#6188,.T.);
#8279=ORIENTED_EDGE('',*,*,#6189,.T.);
#8280=ORIENTED_EDGE('',*,*,#6190,.T.);
#8281=ORIENTED_EDGE('',*,*,#6191,.T.);
#8282=ORIENTED_EDGE('',*,*,#6192,.T.);
#8283=ORIENTED_EDGE('',*,*,#6193,.T.);
#8284=ORIENTED_EDGE('',*,*,#6194,.T.);
#8285=ORIENTED_EDGE('',*,*,#6195,.T.);
#8286=ORIENTED_EDGE('',*,*,#6196,.T.);
#8287=ORIENTED_EDGE('',*,*,#6197,.T.);
#8288=ORIENTED_EDGE('',*,*,#6198,.T.);
#8289=ORIENTED_EDGE('',*,*,#6199,.T.);
#8290=ORIENTED_EDGE('',*,*,#6200,.T.);
#8291=ORIENTED_EDGE('',*,*,#6201,.T.);
#8292=ORIENTED_EDGE('',*,*,#6192,.F.);
#8293=ORIENTED_EDGE('',*,*,#6202,.F.);
#8294=ORIENTED_EDGE('',*,*,#6203,.F.);
#8295=ORIENTED_EDGE('',*,*,#6204,.F.);
#8296=ORIENTED_EDGE('',*,*,#6205,.F.);
#8297=ORIENTED_EDGE('',*,*,#6206,.F.);
#8298=ORIENTED_EDGE('',*,*,#6207,.F.);
#8299=ORIENTED_EDGE('',*,*,#6208,.F.);
#8300=ORIENTED_EDGE('',*,*,#6209,.F.);
#8301=ORIENTED_EDGE('',*,*,#6210,.T.);
#8302=ORIENTED_EDGE('',*,*,#6190,.F.);
#8303=ORIENTED_EDGE('',*,*,#6167,.F.);
#8304=ORIENTED_EDGE('',*,*,#6163,.F.);
#8305=ORIENTED_EDGE('',*,*,#6160,.F.);
#8306=ORIENTED_EDGE('',*,*,#6157,.F.);
#8307=ORIENTED_EDGE('',*,*,#6154,.F.);
#8308=ORIENTED_EDGE('',*,*,#6150,.F.);
#8309=ORIENTED_EDGE('',*,*,#6211,.F.);
#8310=ORIENTED_EDGE('',*,*,#6212,.F.);
#8311=ORIENTED_EDGE('',*,*,#6205,.T.);
#8312=ORIENTED_EDGE('',*,*,#6213,.T.);
#8313=ORIENTED_EDGE('',*,*,#6214,.F.);
#8314=ORIENTED_EDGE('',*,*,#6215,.F.);
#8315=ORIENTED_EDGE('',*,*,#6216,.F.);
#8316=ORIENTED_EDGE('',*,*,#6217,.F.);
#8317=ORIENTED_EDGE('',*,*,#6197,.F.);
#8318=ORIENTED_EDGE('',*,*,#6218,.T.);
#8319=ORIENTED_EDGE('',*,*,#6193,.F.);
#8320=ORIENTED_EDGE('',*,*,#6201,.F.);
#8321=ORIENTED_EDGE('',*,*,#6219,.T.);
#8322=ORIENTED_EDGE('',*,*,#6210,.F.);
#8323=ORIENTED_EDGE('',*,*,#6220,.T.);
#8324=ORIENTED_EDGE('',*,*,#6221,.F.);
#8325=ORIENTED_EDGE('',*,*,#6186,.T.);
#8326=ORIENTED_EDGE('',*,*,#6184,.F.);
#8327=ORIENTED_EDGE('',*,*,#6222,.F.);
#8328=ORIENTED_EDGE('',*,*,#6223,.F.);
#8329=ORIENTED_EDGE('',*,*,#6224,.F.);
#8330=ORIENTED_EDGE('',*,*,#6220,.F.);
#8331=ORIENTED_EDGE('',*,*,#6209,.T.);
#8332=ORIENTED_EDGE('',*,*,#6225,.T.);
#8333=ORIENTED_EDGE('',*,*,#6226,.T.);
#8334=ORIENTED_EDGE('',*,*,#6227,.T.);
#8335=ORIENTED_EDGE('',*,*,#6189,.F.);
#8336=ORIENTED_EDGE('',*,*,#6228,.F.);
#8337=ORIENTED_EDGE('',*,*,#6202,.T.);
#8338=ORIENTED_EDGE('',*,*,#6229,.T.);
#8339=ORIENTED_EDGE('',*,*,#6230,.F.);
#8340=ORIENTED_EDGE('',*,*,#6231,.F.);
#8341=ORIENTED_EDGE('',*,*,#6188,.F.);
#8342=ORIENTED_EDGE('',*,*,#6232,.T.);
#8343=ORIENTED_EDGE('',*,*,#6226,.F.);
#8344=ORIENTED_EDGE('',*,*,#6225,.F.);
#8345=ORIENTED_EDGE('',*,*,#6208,.T.);
#8346=ORIENTED_EDGE('',*,*,#6233,.T.);
#8347=ORIENTED_EDGE('',*,*,#6234,.F.);
#8348=ORIENTED_EDGE('',*,*,#6235,.F.);
#8349=ORIENTED_EDGE('',*,*,#6203,.T.);
#8350=ORIENTED_EDGE('',*,*,#6228,.T.);
#8351=ORIENTED_EDGE('',*,*,#6231,.T.);
#8352=ORIENTED_EDGE('',*,*,#6236,.F.);
#8353=ORIENTED_EDGE('',*,*,#6213,.F.);
#8354=ORIENTED_EDGE('',*,*,#6204,.T.);
#8355=ORIENTED_EDGE('',*,*,#6235,.T.);
#8356=ORIENTED_EDGE('',*,*,#6237,.F.);
#8357=ORIENTED_EDGE('',*,*,#6238,.F.);
#8358=ORIENTED_EDGE('',*,*,#6206,.T.);
#8359=ORIENTED_EDGE('',*,*,#6212,.T.);
#8360=ORIENTED_EDGE('',*,*,#6239,.F.);
#8361=ORIENTED_EDGE('',*,*,#6229,.F.);
#8362=ORIENTED_EDGE('',*,*,#6233,.F.);
#8363=ORIENTED_EDGE('',*,*,#6207,.T.);
#8364=ORIENTED_EDGE('',*,*,#6238,.T.);
#8365=ORIENTED_EDGE('',*,*,#6230,.T.);
#8366=ORIENTED_EDGE('',*,*,#6239,.T.);
#8367=ORIENTED_EDGE('',*,*,#6237,.T.);
#8368=ORIENTED_EDGE('',*,*,#6211,.T.);
#8369=ORIENTED_EDGE('',*,*,#6236,.T.);
#8370=ORIENTED_EDGE('',*,*,#6234,.T.);
#8371=ORIENTED_EDGE('',*,*,#6152,.T.);
#8372=ORIENTED_EDGE('',*,*,#6155,.T.);
#8373=ORIENTED_EDGE('',*,*,#6158,.T.);
#8374=ORIENTED_EDGE('',*,*,#6161,.T.);
#8375=ORIENTED_EDGE('',*,*,#6191,.F.);
#8376=ORIENTED_EDGE('',*,*,#6221,.T.);
#8377=ORIENTED_EDGE('',*,*,#6227,.F.);
#8378=ORIENTED_EDGE('',*,*,#6232,.F.);
#8379=ORIENTED_EDGE('',*,*,#6187,.F.);
#8380=ORIENTED_EDGE('',*,*,#6240,.F.);
#8381=ORIENTED_EDGE('',*,*,#6178,.T.);
#8382=ORIENTED_EDGE('',*,*,#6241,.T.);
#8383=ORIENTED_EDGE('',*,*,#6223,.T.);
#8384=ORIENTED_EDGE('',*,*,#6183,.F.);
#8385=ORIENTED_EDGE('',*,*,#6242,.T.);
#8386=ORIENTED_EDGE('',*,*,#6240,.T.);
#8387=ORIENTED_EDGE('',*,*,#6222,.T.);
#8388=ORIENTED_EDGE('',*,*,#6241,.F.);
#8389=ORIENTED_EDGE('',*,*,#6243,.T.);
#8390=ORIENTED_EDGE('',*,*,#6185,.T.);
#8391=ORIENTED_EDGE('',*,*,#6224,.T.);
#8392=ORIENTED_EDGE('',*,*,#6244,.T.);
#8393=ORIENTED_EDGE('',*,*,#6245,.T.);
#8394=ORIENTED_EDGE('',*,*,#6180,.T.);
#8395=ORIENTED_EDGE('',*,*,#6246,.T.);
#8396=ORIENTED_EDGE('',*,*,#6179,.F.);
#8397=ORIENTED_EDGE('',*,*,#6242,.F.);
#8398=ORIENTED_EDGE('',*,*,#6247,.F.);
#8399=ORIENTED_EDGE('',*,*,#6246,.F.);
#8400=ORIENTED_EDGE('',*,*,#6247,.T.);
#8401=ORIENTED_EDGE('',*,*,#6182,.F.);
#8402=ORIENTED_EDGE('',*,*,#6248,.F.);
#8403=ORIENTED_EDGE('',*,*,#6244,.F.);
#8404=ORIENTED_EDGE('',*,*,#6248,.T.);
#8405=ORIENTED_EDGE('',*,*,#6243,.F.);
#8406=ORIENTED_EDGE('',*,*,#6181,.T.);
#8407=ORIENTED_EDGE('',*,*,#6245,.F.);
#8408=ORIENTED_EDGE('',*,*,#6249,.F.);
#8409=ORIENTED_EDGE('',*,*,#6169,.T.);
#8410=ORIENTED_EDGE('',*,*,#6177,.T.);
#8411=ORIENTED_EDGE('',*,*,#6250,.F.);
#8412=ORIENTED_EDGE('',*,*,#6173,.T.);
#8413=ORIENTED_EDGE('',*,*,#6175,.T.);
#8414=ORIENTED_EDGE('',*,*,#6251,.T.);
#8415=ORIENTED_EDGE('',*,*,#6250,.T.);
#8416=ORIENTED_EDGE('',*,*,#6176,.F.);
#8417=ORIENTED_EDGE('',*,*,#6251,.F.);
#8418=ORIENTED_EDGE('',*,*,#6174,.F.);
#8419=ORIENTED_EDGE('',*,*,#6171,.T.);
#8420=ORIENTED_EDGE('',*,*,#6252,.T.);
#8421=ORIENTED_EDGE('',*,*,#6249,.T.);
#8422=ORIENTED_EDGE('',*,*,#6172,.F.);
#8423=ORIENTED_EDGE('',*,*,#6252,.F.);
#8424=ORIENTED_EDGE('',*,*,#6170,.F.);
#8425=ORIENTED_EDGE('',*,*,#6253,.T.);
#8426=ORIENTED_EDGE('',*,*,#6198,.F.);
#8427=ORIENTED_EDGE('',*,*,#6219,.F.);
#8428=ORIENTED_EDGE('',*,*,#6200,.F.);
#8429=ORIENTED_EDGE('',*,*,#6253,.F.);
#8430=ORIENTED_EDGE('',*,*,#6199,.F.);
#8431=ORIENTED_EDGE('',*,*,#6254,.T.);
#8432=ORIENTED_EDGE('',*,*,#6194,.F.);
#8433=ORIENTED_EDGE('',*,*,#6218,.F.);
#8434=ORIENTED_EDGE('',*,*,#6196,.F.);
#8435=ORIENTED_EDGE('',*,*,#6254,.F.);
#8436=ORIENTED_EDGE('',*,*,#6195,.F.);
#8437=ORIENTED_EDGE('',*,*,#6215,.T.);
#8438=ORIENTED_EDGE('',*,*,#6255,.F.);
#8439=ORIENTED_EDGE('',*,*,#6256,.F.);
#8440=ORIENTED_EDGE('',*,*,#6257,.T.);
#8441=ORIENTED_EDGE('',*,*,#6164,.F.);
#8442=ORIENTED_EDGE('',*,*,#6214,.T.);
#8443=ORIENTED_EDGE('',*,*,#6258,.F.);
#8444=ORIENTED_EDGE('',*,*,#6259,.F.);
#8445=ORIENTED_EDGE('',*,*,#6255,.T.);
#8446=ORIENTED_EDGE('',*,*,#6217,.T.);
#8447=ORIENTED_EDGE('',*,*,#6260,.F.);
#8448=ORIENTED_EDGE('',*,*,#6261,.F.);
#8449=ORIENTED_EDGE('',*,*,#6258,.T.);
#8450=ORIENTED_EDGE('',*,*,#6166,.F.);
#8451=ORIENTED_EDGE('',*,*,#6216,.T.);
#8452=ORIENTED_EDGE('',*,*,#6257,.F.);
#8453=ORIENTED_EDGE('',*,*,#6262,.F.);
#8454=ORIENTED_EDGE('',*,*,#6260,.T.);
#8455=ORIENTED_EDGE('',*,*,#6256,.T.);
#8456=ORIENTED_EDGE('',*,*,#6259,.T.);
#8457=ORIENTED_EDGE('',*,*,#6261,.T.);
#8458=ORIENTED_EDGE('',*,*,#6262,.T.);
#8459=ORIENTED_EDGE('',*,*,#6146,.T.);
#10229=CYLINDRICAL_SURFACE('',#11584,2.);
#10230=CYLINDRICAL_SURFACE('',#11586,1.);
#10231=CYLINDRICAL_SURFACE('',#11589,1.);
#10232=CYLINDRICAL_SURFACE('',#11592,1.5);
#10233=CYLINDRICAL_SURFACE('',#11595,1.5);
#10234=CYLINDRICAL_SURFACE('',#11598,1.);
#10235=CYLINDRICAL_SURFACE('',#11601,2.75);
#10236=CYLINDRICAL_SURFACE('',#11611,10.2500000000004);
#10237=CYLINDRICAL_SURFACE('',#11614,11.25);
#10238=CYLINDRICAL_SURFACE('',#11618,2.75);
#10239=CYLINDRICAL_SURFACE('',#11633,11.25);
#10240=CYLINDRICAL_SURFACE('',#11640,3.);
#10241=CYLINDRICAL_SURFACE('',#11642,3.);
#10242=CYLINDRICAL_SURFACE('',#11647,10.2500000000004);
#10243=CYLINDRICAL_SURFACE('',#11652,1.5);
#10244=CYLINDRICAL_SURFACE('',#11654,1.5);
#10591=ADVANCED_FACE('',(#954),#154,.T.);
#10592=ADVANCED_FACE('',(#955),#10229,.T.);
#10593=ADVANCED_FACE('',(#956),#10230,.F.);
#10594=ADVANCED_FACE('',(#957),#10231,.F.);
#10595=ADVANCED_FACE('',(#958),#10232,.F.);
#10596=ADVANCED_FACE('',(#959),#10233,.F.);
#10597=ADVANCED_FACE('',(#960),#10234,.F.);
#10598=ADVANCED_FACE('',(#961),#10235,.T.);
#10599=ADVANCED_FACE('',(#962),#155,.T.);
#10600=ADVANCED_FACE('',(#963),#10236,.T.);
#10601=ADVANCED_FACE('',(#964),#10237,.T.);
#10602=ADVANCED_FACE('',(#965),#10238,.T.);
#10603=ADVANCED_FACE('',(#966,#327,#328,#329,#330,#331,#332),#523,.F.);
#10604=ADVANCED_FACE('',(#967,#333),#524,.T.);
#10605=ADVANCED_FACE('',(#968),#525,.T.);
#10606=ADVANCED_FACE('',(#969,#334),#526,.T.);
#10607=ADVANCED_FACE('',(#970),#10239,.T.);
#10608=ADVANCED_FACE('',(#971),#527,.T.);
#10609=ADVANCED_FACE('',(#972),#528,.T.);
#10610=ADVANCED_FACE('',(#973),#529,.T.);
#10611=ADVANCED_FACE('',(#974),#530,.T.);
#10612=ADVANCED_FACE('',(#975),#10240,.T.);
#10613=ADVANCED_FACE('',(#976),#10241,.T.);
#10614=ADVANCED_FACE('',(#977),#531,.T.);
#10615=ADVANCED_FACE('',(#978,#335,#336,#337,#338,#339),#532,.T.);
#10616=ADVANCED_FACE('',(#979),#533,.F.);
#10617=ADVANCED_FACE('',(#980),#10242,.T.);
#10618=ADVANCED_FACE('',(#981),#534,.F.);
#10619=ADVANCED_FACE('',(#982),#535,.F.);
#10620=ADVANCED_FACE('',(#983),#536,.T.);
#10621=ADVANCED_FACE('',(#984),#10243,.T.);
#10622=ADVANCED_FACE('',(#985),#156,.T.);
#10623=ADVANCED_FACE('',(#986),#10244,.T.);
#10624=ADVANCED_FACE('',(#987),#537,.T.);
#10625=ADVANCED_FACE('',(#988),#538,.T.);
#10626=ADVANCED_FACE('',(#989),#539,.F.);
#10627=ADVANCED_FACE('',(#990),#540,.T.);
#10628=ADVANCED_FACE('',(#991),#541,.F.);
#10629=ADVANCED_FACE('',(#992),#542,.T.);
#10630=ADVANCED_FACE('',(#993),#543,.T.);
#10631=ADVANCED_FACE('',(#994),#544,.T.);
#10632=ADVANCED_FACE('',(#995),#545,.T.);
#10633=ADVANCED_FACE('',(#996,#340),#546,.F.);
#10634=ADVANCED_FACE('',(#997),#547,.F.);
#10635=ADVANCED_FACE('',(#998,#341),#548,.F.);
#10636=ADVANCED_FACE('',(#999),#549,.F.);
#10637=ADVANCED_FACE('',(#1000),#550,.T.);
#10638=ADVANCED_FACE('',(#1001),#551,.T.);
#10965=CLOSED_SHELL('',(#10591,#10592,#10593,#10594,#10595,#10596,#10597,
#10598,#10599,#10600,#10601,#10602,#10603,#10604,#10605,#10606,#10607,#10608,
#10609,#10610,#10611,#10612,#10613,#10614,#10615,#10616,#10617,#10618,#10619,
#10620,#10621,#10622,#10623,#10624,#10625,#10626,#10627,#10628,#10629,#10630,
#10631,#10632,#10633,#10634,#10635,#10636,#10637,#10638));
#11578=AXIS2_PLACEMENT_3D('',#16771,#13518,#13519);
#11579=AXIS2_PLACEMENT_3D('',#16772,#13520,#13521);
#11580=AXIS2_PLACEMENT_3D('',#16774,#13522,#13523);
#11581=AXIS2_PLACEMENT_3D('',#16776,#13524,#13525);
#11582=AXIS2_PLACEMENT_3D('',#16778,#13526,#13527);
#11583=AXIS2_PLACEMENT_3D('',#16779,#13528,#13529);
#11584=AXIS2_PLACEMENT_3D('',#16780,#13530,#13531);
#11585=AXIS2_PLACEMENT_3D('',#16782,#13532,#13533);
#11586=AXIS2_PLACEMENT_3D('',#16784,#13535,#13536);
#11587=AXIS2_PLACEMENT_3D('',#16786,#13537,#13538);
#11588=AXIS2_PLACEMENT_3D('',#16789,#13540,#13541);
#11589=AXIS2_PLACEMENT_3D('',#16790,#13542,#13543);
#11590=AXIS2_PLACEMENT_3D('',#16792,#13544,#13545);
#11591=AXIS2_PLACEMENT_3D('',#16795,#13547,#13548);
#11592=AXIS2_PLACEMENT_3D('',#16796,#13549,#13550);
#11593=AXIS2_PLACEMENT_3D('',#16798,#13551,#13552);
#11594=AXIS2_PLACEMENT_3D('',#16801,#13554,#13555);
#11595=AXIS2_PLACEMENT_3D('',#16802,#13556,#13557);
#11596=AXIS2_PLACEMENT_3D('',#16804,#13558,#13559);
#11597=AXIS2_PLACEMENT_3D('',#16807,#13561,#13562);
#11598=AXIS2_PLACEMENT_3D('',#16808,#13563,#13564);
#11599=AXIS2_PLACEMENT_3D('',#16810,#13565,#13566);
#11600=AXIS2_PLACEMENT_3D('',#16813,#13568,#13569);
#11601=AXIS2_PLACEMENT_3D('',#16814,#13570,#13571);
#11602=AXIS2_PLACEMENT_3D('',#16816,#13572,#13573);
#11603=AXIS2_PLACEMENT_3D('',#16820,#13575,#13576);
#11604=AXIS2_PLACEMENT_3D('',#16824,#13578,#13579);
#11605=AXIS2_PLACEMENT_3D('',#16828,#13581,#13582);
#11606=AXIS2_PLACEMENT_3D('',#16832,#13584,#13585);
#11607=AXIS2_PLACEMENT_3D('',#16835,#13587,#13588);
#11608=AXIS2_PLACEMENT_3D('',#16836,#13589,#13590);
#11609=AXIS2_PLACEMENT_3D('',#16839,#13591,#13592);
#11610=AXIS2_PLACEMENT_3D('',#16856,#13593,#13594);
#11611=AXIS2_PLACEMENT_3D('',#16871,#13595,#13596);
#11612=AXIS2_PLACEMENT_3D('',#16874,#13597,#13598);
#11613=AXIS2_PLACEMENT_3D('',#16878,#13600,#13601);
#11614=AXIS2_PLACEMENT_3D('',#16880,#13603,#13604);
#11615=AXIS2_PLACEMENT_3D('',#16883,#13605,#13606);
#11616=AXIS2_PLACEMENT_3D('',#16887,#13608,#13609);
#11617=AXIS2_PLACEMENT_3D('',#16889,#13610,#13611);
#11618=AXIS2_PLACEMENT_3D('',#16891,#13613,#13614);
#11619=AXIS2_PLACEMENT_3D('',#16893,#13615,#13616);
#11620=AXIS2_PLACEMENT_3D('',#16897,#13618,#13619);
#11621=AXIS2_PLACEMENT_3D('',#16901,#13621,#13622);
#11622=AXIS2_PLACEMENT_3D('',#16905,#13624,#13625);
#11623=AXIS2_PLACEMENT_3D('',#16909,#13627,#13628);
#11624=AXIS2_PLACEMENT_3D('',#16912,#13630,#13631);
#11625=AXIS2_PLACEMENT_3D('',#16913,#13632,#13633);
#11626=AXIS2_PLACEMENT_3D('',#16919,#13636,#13637);
#11627=AXIS2_PLACEMENT_3D('',#16923,#13639,#13640);
#11628=AXIS2_PLACEMENT_3D('',#16931,#13645,#13646);
#11629=AXIS2_PLACEMENT_3D('',#16945,#13654,#13655);
#11630=AXIS2_PLACEMENT_3D('',#16948,#13658,#13659);
#11631=AXIS2_PLACEMENT_3D('',#16950,#13660,#13661);
#11632=AXIS2_PLACEMENT_3D('',#16955,#13664,#13665);
#11633=AXIS2_PLACEMENT_3D('',#16957,#13667,#13668);
#11634=AXIS2_PLACEMENT_3D('',#16959,#13669,#13670);
#11635=AXIS2_PLACEMENT_3D('',#16961,#13671,#13672);
#11636=AXIS2_PLACEMENT_3D('',#16963,#13674,#13675);
#11637=AXIS2_PLACEMENT_3D('',#16965,#13677,#13678);
#11638=AXIS2_PLACEMENT_3D('',#16972,#13683,#13684);
#11639=AXIS2_PLACEMENT_3D('',#16974,#13686,#13687);
#11640=AXIS2_PLACEMENT_3D('',#16978,#13690,#13691);
#11641=AXIS2_PLACEMENT_3D('',#16979,#13692,#13693);
#11642=AXIS2_PLACEMENT_3D('',#16980,#13694,#13695);
#11643=AXIS2_PLACEMENT_3D('',#16982,#13696,#13697);
#11644=AXIS2_PLACEMENT_3D('',#16984,#13699,#13700);
#11645=AXIS2_PLACEMENT_3D('',#16986,#13702,#13703);
#11646=AXIS2_PLACEMENT_3D('',#16987,#13704,#13705);
#11647=AXIS2_PLACEMENT_3D('',#16988,#13706,#13707);
#11648=AXIS2_PLACEMENT_3D('',#16991,#13710,#13711);
#11649=AXIS2_PLACEMENT_3D('',#16993,#13713,#13714);
#11650=AXIS2_PLACEMENT_3D('',#16995,#13716,#13717);
#11651=AXIS2_PLACEMENT_3D('',#16998,#13718,#13719);
#11652=AXIS2_PLACEMENT_3D('',#17001,#13722,#13723);
#11653=AXIS2_PLACEMENT_3D('',#17016,#13724,#13725);
#11654=AXIS2_PLACEMENT_3D('',#17031,#13726,#13727);
#11655=AXIS2_PLACEMENT_3D('',#17032,#13728,#13729);
#11656=AXIS2_PLACEMENT_3D('',#17035,#13732,#13733);
#11657=AXIS2_PLACEMENT_3D('',#17037,#13735,#13736);
#11658=AXIS2_PLACEMENT_3D('',#17038,#13737,#13738);
#11659=AXIS2_PLACEMENT_3D('',#17040,#13740,#13741);
#11660=AXIS2_PLACEMENT_3D('',#17041,#13742,#13743);
#11661=AXIS2_PLACEMENT_3D('',#17043,#13745,#13746);
#11662=AXIS2_PLACEMENT_3D('',#17044,#13747,#13748);
#11663=AXIS2_PLACEMENT_3D('',#17046,#13750,#13751);
#11664=AXIS2_PLACEMENT_3D('',#17047,#13752,#13753);
#11665=AXIS2_PLACEMENT_3D('',#17053,#13757,#13758);
#11666=AXIS2_PLACEMENT_3D('',#17057,#13761,#13762);
#11667=AXIS2_PLACEMENT_3D('',#17061,#13765,#13766);
#11668=AXIS2_PLACEMENT_3D('',#17063,#13768,#13769);
#11669=AXIS2_PLACEMENT_3D('',#17064,#13770,#13771);
#13518=DIRECTION('axis',(0.,0.,1.));
#13519=DIRECTION('refdir',(1.,0.,0.));
#13520=DIRECTION('center_axis',(0.,0.,-1.));
#13521=DIRECTION('ref_axis',(-1.,0.,0.));
#13522=DIRECTION('center_axis',(0.,0.,-1.));
#13523=DIRECTION('ref_axis',(-1.,0.,0.));
#13524=DIRECTION('center_axis',(0.,-1.,0.));
#13525=DIRECTION('ref_axis',(1.,0.,0.));
#13526=DIRECTION('center_axis',(0.,0.,1.));
#13527=DIRECTION('ref_axis',(-1.,0.,0.));
#13528=DIRECTION('center_axis',(0.,0.,1.));
#13529=DIRECTION('ref_axis',(-1.,0.,0.));
#13530=DIRECTION('center_axis',(0.,0.,1.));
#13531=DIRECTION('ref_axis',(1.,0.,0.));
#13532=DIRECTION('center_axis',(0.,0.,-1.));
#13533=DIRECTION('ref_axis',(1.,0.,0.));
#13534=DIRECTION('',(0.,0.,-1.));
#13535=DIRECTION('center_axis',(0.,0.,-1.));
#13536=DIRECTION('ref_axis',(-1.,0.,0.));
#13537=DIRECTION('center_axis',(0.,0.,-1.));
#13538=DIRECTION('ref_axis',(1.,0.,0.));
#13539=DIRECTION('',(0.,0.,-1.));
#13540=DIRECTION('center_axis',(0.,0.,-1.));
#13541=DIRECTION('ref_axis',(-1.,0.,0.));
#13542=DIRECTION('center_axis',(0.,0.,-1.));
#13543=DIRECTION('ref_axis',(-1.,0.,0.));
#13544=DIRECTION('center_axis',(0.,0.,-1.));
#13545=DIRECTION('ref_axis',(1.,0.,0.));
#13546=DIRECTION('',(0.,0.,-1.));
#13547=DIRECTION('center_axis',(0.,0.,-1.));
#13548=DIRECTION('ref_axis',(-1.,0.,0.));
#13549=DIRECTION('center_axis',(0.,0.,-1.));
#13550=DIRECTION('ref_axis',(-1.,0.,0.));
#13551=DIRECTION('center_axis',(0.,0.,-1.));
#13552=DIRECTION('ref_axis',(1.,0.,0.));
#13553=DIRECTION('',(0.,0.,-1.));
#13554=DIRECTION('center_axis',(0.,0.,-1.));
#13555=DIRECTION('ref_axis',(-1.,0.,0.));
#13556=DIRECTION('center_axis',(0.,0.,-1.));
#13557=DIRECTION('ref_axis',(-1.,0.,0.));
#13558=DIRECTION('center_axis',(0.,0.,-1.));
#13559=DIRECTION('ref_axis',(1.,0.,0.));
#13560=DIRECTION('',(0.,0.,-1.));
#13561=DIRECTION('center_axis',(0.,0.,-1.));
#13562=DIRECTION('ref_axis',(-1.,0.,0.));
#13563=DIRECTION('center_axis',(0.,0.,1.));
#13564=DIRECTION('ref_axis',(1.,0.,0.));
#13565=DIRECTION('center_axis',(0.,0.,-1.));
#13566=DIRECTION('ref_axis',(1.,0.,0.));
#13567=DIRECTION('',(0.,0.,1.));
#13568=DIRECTION('center_axis',(0.,0.,1.));
#13569=DIRECTION('ref_axis',(1.,0.,0.));
#13570=DIRECTION('center_axis',(0.,0.,1.));
#13571=DIRECTION('ref_axis',(1.,0.,0.));
#13572=DIRECTION('center_axis',(0.,0.,-1.));
#13573=DIRECTION('ref_axis',(1.,0.,0.));
#13574=DIRECTION('',(0.,0.,-1.));
#13575=DIRECTION('center_axis',(0.,0.,-1.));
#13576=DIRECTION('ref_axis',(-1.,0.,0.));
#13577=DIRECTION('',(0.,0.,1.));
#13578=DIRECTION('center_axis',(0.,0.,-1.));
#13579=DIRECTION('ref_axis',(-1.,0.,0.));
#13580=DIRECTION('',(0.,0.,-1.));
#13581=DIRECTION('center_axis',(0.,0.,-1.));
#13582=DIRECTION('ref_axis',(-1.,0.,0.));
#13583=DIRECTION('',(0.,0.,1.));
#13584=DIRECTION('center_axis',(0.,0.,-1.));
#13585=DIRECTION('ref_axis',(-1.,0.,0.));
#13586=DIRECTION('',(0.,0.,-1.));
#13587=DIRECTION('center_axis',(0.,0.,-1.));
#13588=DIRECTION('ref_axis',(-1.,0.,0.));
#13589=DIRECTION('center_axis',(1.,3.08395284618099E-16,0.));
#13590=DIRECTION('ref_axis',(0.,1.,0.));
#13591=DIRECTION('center_axis',(-1.,0.,0.));
#13592=DIRECTION('ref_axis',(0.,1.,0.));
#13593=DIRECTION('center_axis',(1.,0.,0.));
#13594=DIRECTION('ref_axis',(0.,1.,0.));
#13595=DIRECTION('center_axis',(-1.,0.,0.));
#13596=DIRECTION('ref_axis',(0.,-1.,0.));
#13597=DIRECTION('center_axis',(-1.,-8.83324975243572E-46,5.21932234251264E-31));
#13598=DIRECTION('ref_axis',(-7.64335950198467E-61,1.,1.69241314729438E-15));
#13599=DIRECTION('',(-1.,-3.08395284618099E-16,0.));
#13600=DIRECTION('center_axis',(1.,0.,0.));
#13601=DIRECTION('ref_axis',(0.,1.,0.));
#13602=DIRECTION('',(-1.,-3.08395284618099E-16,0.));
#13603=DIRECTION('center_axis',(-1.,0.,0.));
#13604=DIRECTION('ref_axis',(0.,-1.,0.));
#13605=DIRECTION('center_axis',(1.,0.,0.));
#13606=DIRECTION('ref_axis',(0.,1.,0.));
#13607=DIRECTION('',(-1.,-3.08395284618099E-16,0.));
#13608=DIRECTION('center_axis',(1.,0.,0.));
#13609=DIRECTION('ref_axis',(0.,1.,0.));
#13610=DIRECTION('center_axis',(1.,0.,0.));
#13611=DIRECTION('ref_axis',(0.,1.,0.));
#13612=DIRECTION('',(1.,3.08395284618099E-16,0.));
#13613=DIRECTION('center_axis',(0.,0.,-1.));
#13614=DIRECTION('ref_axis',(-1.,0.,0.));
#13615=DIRECTION('center_axis',(0.,0.,1.));
#13616=DIRECTION('ref_axis',(1.,0.,0.));
#13617=DIRECTION('',(0.,0.,1.));
#13618=DIRECTION('center_axis',(0.,0.,-1.));
#13619=DIRECTION('ref_axis',(-1.,0.,0.));
#13620=DIRECTION('',(0.,0.,-1.));
#13621=DIRECTION('center_axis',(0.,0.,-1.));
#13622=DIRECTION('ref_axis',(1.,6.30808536718839E-16,0.));
#13623=DIRECTION('',(0.,0.,1.));
#13624=DIRECTION('center_axis',(0.,0.,-1.));
#13625=DIRECTION('ref_axis',(-1.,0.,0.));
#13626=DIRECTION('',(0.,0.,-1.));
#13627=DIRECTION('center_axis',(0.,0.,-1.));
#13628=DIRECTION('ref_axis',(1.,6.30808536718839E-16,0.));
#13629=DIRECTION('',(0.,0.,1.));
#13630=DIRECTION('center_axis',(0.,0.,-1.));
#13631=DIRECTION('ref_axis',(-1.,0.,0.));
#13632=DIRECTION('center_axis',(0.,0.,1.));
#13633=DIRECTION('ref_axis',(1.,0.,0.));
#13634=DIRECTION('',(-3.08395284618099E-16,1.,0.));
#13635=DIRECTION('',(1.,0.,0.));
#13636=DIRECTION('center_axis',(0.,0.,1.));
#13637=DIRECTION('ref_axis',(-1.,0.,0.));
#13638=DIRECTION('',(0.,-1.,0.));
#13639=DIRECTION('center_axis',(0.,0.,1.));
#13640=DIRECTION('ref_axis',(1.,0.,0.));
#13641=DIRECTION('',(-1.,0.,0.));
#13642=DIRECTION('',(-3.08395284618099E-16,1.,0.));
#13643=DIRECTION('',(-1.,-3.08395284618099E-16,0.));
#13644=DIRECTION('',(3.09492820192543E-16,-1.,0.));
#13645=DIRECTION('center_axis',(-1.,0.,0.));
#13646=DIRECTION('ref_axis',(0.,0.,1.));
#13647=DIRECTION('',(0.,-1.,0.));
#13648=DIRECTION('',(0.,0.,1.));
#13649=DIRECTION('',(0.,0.,1.));
#13650=DIRECTION('',(0.,0.,1.));
#13651=DIRECTION('',(0.,-1.,0.));
#13652=DIRECTION('',(0.,0.,-1.));
#13653=DIRECTION('',(0.,1.,-3.46944695195362E-16));
#13654=DIRECTION('center_axis',(0.,0.,1.));
#13655=DIRECTION('ref_axis',(1.,0.,0.));
#13656=DIRECTION('',(1.,0.,0.));
#13657=DIRECTION('',(-1.,0.,0.));
#13658=DIRECTION('center_axis',(1.,2.93307512767319E-47,9.51076515746783E-32));
#13659=DIRECTION('ref_axis',(8.86148785842978E-64,1.,-3.08395284618099E-16));
#13660=DIRECTION('center_axis',(1.,0.,0.));
#13661=DIRECTION('ref_axis',(0.,1.,0.));
#13662=DIRECTION('',(-3.01691039300315E-16,1.,0.));
#13663=DIRECTION('',(4.96586290813306E-16,-1.,0.));
#13664=DIRECTION('center_axis',(1.,0.,0.));
#13665=DIRECTION('ref_axis',(0.,1.,0.));
#13666=DIRECTION('',(-5.41424068523692E-16,1.,0.));
#13667=DIRECTION('center_axis',(-1.,0.,0.));
#13668=DIRECTION('ref_axis',(0.,0.998520612789804,-0.0543744961712152));
#13669=DIRECTION('center_axis',(1.,0.,0.));
#13670=DIRECTION('ref_axis',(0.,1.,0.));
#13671=DIRECTION('center_axis',(1.,0.,0.));
#13672=DIRECTION('ref_axis',(0.,1.,0.));
#13673=DIRECTION('',(1.,3.08395284618099E-16,0.));
#13674=DIRECTION('center_axis',(1.,2.93307512767319E-47,9.51076515746783E-32));
#13675=DIRECTION('ref_axis',(8.86148785842978E-64,1.,-3.08395284618099E-16));
#13676=DIRECTION('',(0.,0.,1.));
#13677=DIRECTION('center_axis',(1.,2.93307512767319E-47,9.51076515746783E-32));
#13678=DIRECTION('ref_axis',(8.86148785842978E-64,1.,-3.08395284618099E-16));
#13679=DIRECTION('',(0.,0.,1.));
#13680=DIRECTION('',(-3.08395284618099E-16,1.,0.));
#13681=DIRECTION('',(0.,0.,1.));
#13682=DIRECTION('',(-3.01691039300315E-16,1.,0.));
#13683=DIRECTION('center_axis',(1.,2.93307512767319E-47,9.51076515746783E-32));
#13684=DIRECTION('ref_axis',(8.86148785842978E-64,1.,-3.08395284618099E-16));
#13685=DIRECTION('',(0.,0.,1.));
#13686=DIRECTION('center_axis',(0.,-1.,0.));
#13687=DIRECTION('ref_axis',(0.,0.,-1.));
#13688=DIRECTION('',(1.,0.,0.));
#13689=DIRECTION('',(0.,0.,1.));
#13690=DIRECTION('center_axis',(0.,0.,1.));
#13691=DIRECTION('ref_axis',(1.,0.,0.));
#13692=DIRECTION('center_axis',(0.,0.,1.));
#13693=DIRECTION('ref_axis',(-1.,0.,0.));
#13694=DIRECTION('center_axis',(0.,0.,1.));
#13695=DIRECTION('ref_axis',(1.,0.,0.));
#13696=DIRECTION('center_axis',(0.,0.,1.));
#13697=DIRECTION('ref_axis',(1.,0.,0.));
#13698=DIRECTION('',(0.,0.,1.));
#13699=DIRECTION('center_axis',(0.,1.,0.));
#13700=DIRECTION('ref_axis',(1.,0.,0.));
#13701=DIRECTION('',(-1.,0.,0.));
#13702=DIRECTION('center_axis',(0.,0.,1.));
#13703=DIRECTION('ref_axis',(1.,0.,0.));
#13704=DIRECTION('center_axis',(0.,0.,-1.));
#13705=DIRECTION('ref_axis',(0.,-1.,0.));
#13706=DIRECTION('center_axis',(-1.,0.,0.));
#13707=DIRECTION('ref_axis',(0.,0.999304019410872,-0.0373025037936587));
#13708=DIRECTION('',(-1.,-3.08395284618099E-16,0.));
#13709=DIRECTION('',(-1.,-3.08395284618099E-16,0.));
#13710=DIRECTION('center_axis',(0.,0.,-1.));
#13711=DIRECTION('ref_axis',(0.,-1.,0.));
#13712=DIRECTION('',(-3.08395284618099E-16,1.,0.));
#13713=DIRECTION('center_axis',(0.,0.,1.));
#13714=DIRECTION('ref_axis',(1.,0.,0.));
#13715=DIRECTION('',(3.08395284618099E-16,-1.,0.));
#13716=DIRECTION('center_axis',(1.,2.93307512767319E-47,9.51076515746783E-32));
#13717=DIRECTION('ref_axis',(8.86148785842978E-64,1.,-3.08395284618099E-16));
#13718=DIRECTION('center_axis',(1.,0.,0.));
#13719=DIRECTION('ref_axis',(0.,1.,0.));
#13720=DIRECTION('',(-3.08395284618099E-16,1.,0.));
#13721=DIRECTION('',(3.08395284618099E-16,-1.,0.));
#13722=DIRECTION('center_axis',(0.,1.,0.));
#13723=DIRECTION('ref_axis',(-1.,0.,0.));
#13724=DIRECTION('center_axis',(1.,3.08395284618099E-16,0.));
#13725=DIRECTION('ref_axis',(0.,-0.999304019410872,-0.0373025037936637));
#13726=DIRECTION('center_axis',(0.,-1.,0.));
#13727=DIRECTION('ref_axis',(1.,0.,0.));
#13728=DIRECTION('center_axis',(0.,0.,-1.));
#13729=DIRECTION('ref_axis',(0.,-1.,0.));
#13730=DIRECTION('',(1.,0.,0.));
#13731=DIRECTION('',(-1.,0.,0.));
#13732=DIRECTION('center_axis',(0.,0.,-1.));
#13733=DIRECTION('ref_axis',(0.,-1.,0.));
#13734=DIRECTION('',(-1.,0.,0.));
#13735=DIRECTION('center_axis',(0.,-1.,0.));
#13736=DIRECTION('ref_axis',(0.,0.,-1.));
#13737=DIRECTION('center_axis',(0.,0.,-1.));
#13738=DIRECTION('ref_axis',(0.,-1.,0.));
#13739=DIRECTION('',(1.,0.,0.));
#13740=DIRECTION('center_axis',(0.,1.,0.));
#13741=DIRECTION('ref_axis',(1.,0.,0.));
#13742=DIRECTION('center_axis',(0.,1.,0.));
#13743=DIRECTION('ref_axis',(1.,0.,0.));
#13744=DIRECTION('',(-1.,0.,0.));
#13745=DIRECTION('center_axis',(0.,0.,1.));
#13746=DIRECTION('ref_axis',(1.,0.,0.));
#13747=DIRECTION('center_axis',(0.,-1.,0.));
#13748=DIRECTION('ref_axis',(0.,0.,-1.));
#13749=DIRECTION('',(1.,0.,0.));
#13750=DIRECTION('center_axis',(0.,0.,1.));
#13751=DIRECTION('ref_axis',(1.,0.,0.));
#13752=DIRECTION('center_axis',(0.,0.,1.));
#13753=DIRECTION('ref_axis',(1.,0.,0.));
#13754=DIRECTION('',(1.,0.,0.));
#13755=DIRECTION('',(0.,-1.,0.));
#13756=DIRECTION('',(1.,0.,0.));
#13757=DIRECTION('center_axis',(0.,1.,0.));
#13758=DIRECTION('ref_axis',(1.,0.,0.));
#13759=DIRECTION('',(1.,0.,0.));
#13760=DIRECTION('',(0.,0.,1.));
#13761=DIRECTION('center_axis',(0.,-3.46944695195362E-16,-1.));
#13762=DIRECTION('ref_axis',(0.,-1.,3.46944695195362E-16));
#13763=DIRECTION('',(1.,0.,0.));
#13764=DIRECTION('',(0.,1.,-3.46944695195362E-16));
#13765=DIRECTION('center_axis',(0.,-1.,0.));
#13766=DIRECTION('ref_axis',(0.,0.,-1.));
#13767=DIRECTION('',(0.,0.,-1.));
#13768=DIRECTION('center_axis',(-1.,0.,0.));
#13769=DIRECTION('ref_axis',(0.,0.,1.));
#13770=DIRECTION('center_axis',(0.,0.,-1.));
#13771=DIRECTION('ref_axis',(0.,-1.,0.));
#16771=CARTESIAN_POINT('',(0.,0.,0.));
#16772=CARTESIAN_POINT('Origin',(22.,11.3156378831472,-20.3));
#16773=CARTESIAN_POINT('',(23.8,11.3156378831472,-20.5));
#16774=CARTESIAN_POINT('Origin',(22.,11.3156378831472,-20.5));
#16775=CARTESIAN_POINT('',(24.,11.3156378831472,-20.3));
#16776=CARTESIAN_POINT('Origin',(23.8,11.3156378831472,-20.3));
#16777=CARTESIAN_POINT('',(20.,11.3156378831472,-20.3));
#16778=CARTESIAN_POINT('Origin',(22.,11.3156378831472,-20.3));
#16779=CARTESIAN_POINT('Origin',(22.,11.3156378831472,-20.3));
#16780=CARTESIAN_POINT('Origin',(22.,11.3156378831472,-20.5));
#16781=CARTESIAN_POINT('',(20.,11.3156378831472,-18.5));
#16782=CARTESIAN_POINT('Origin',(22.,11.3156378831472,-18.5));
#16783=CARTESIAN_POINT('',(20.,11.3156378831472,-20.5));
#16784=CARTESIAN_POINT('Origin',(35.,2.,4.24264068711929));
#16785=CARTESIAN_POINT('',(36.,2.,0.));
#16786=CARTESIAN_POINT('Origin',(35.,2.,0.));
#16787=CARTESIAN_POINT('',(36.,2.,-18.5));
#16788=CARTESIAN_POINT('',(36.,2.,4.24264068711929));
#16789=CARTESIAN_POINT('Origin',(35.,2.,-18.5));
#16790=CARTESIAN_POINT('Origin',(35.,20.5,4.24264068711929));
#16791=CARTESIAN_POINT('',(36.,20.5,0.));
#16792=CARTESIAN_POINT('Origin',(35.,20.5,0.));
#16793=CARTESIAN_POINT('',(36.,20.5,-18.5));
#16794=CARTESIAN_POINT('',(36.,20.5,4.24264068711929));
#16795=CARTESIAN_POINT('Origin',(35.,20.5,-18.5));
#16796=CARTESIAN_POINT('Origin',(31.5,2.,4.24264068711929));
#16797=CARTESIAN_POINT('',(33.,2.,0.));
#16798=CARTESIAN_POINT('Origin',(31.5,2.,0.));
#16799=CARTESIAN_POINT('',(33.,2.,-18.5));
#16800=CARTESIAN_POINT('',(33.,2.,4.24264068711929));
#16801=CARTESIAN_POINT('Origin',(31.5,2.,-18.5));
#16802=CARTESIAN_POINT('Origin',(31.5,20.5,4.24264068711929));
#16803=CARTESIAN_POINT('',(33.,20.5,0.));
#16804=CARTESIAN_POINT('Origin',(31.5,20.5,0.));
#16805=CARTESIAN_POINT('',(33.,20.5,-18.5));
#16806=CARTESIAN_POINT('',(33.,20.5,4.24264068711929));
#16807=CARTESIAN_POINT('Origin',(31.5,20.5,-18.5));
#16808=CARTESIAN_POINT('Origin',(-2.25,11.5,-28.501));
#16809=CARTESIAN_POINT('',(-3.25,11.5,-10.75));
#16810=CARTESIAN_POINT('Origin',(-2.25,11.5,-10.75));
#16811=CARTESIAN_POINT('',(-3.25,11.5,-7.75));
#16812=CARTESIAN_POINT('',(-3.25,11.5,-28.501));
#16813=CARTESIAN_POINT('Origin',(-2.25,11.5,-7.75));
#16814=CARTESIAN_POINT('Origin',(11.25,11.3156378831472,-28.5));
#16815=CARTESIAN_POINT('',(8.5,11.3156378831472,-18.5));
#16816=CARTESIAN_POINT('Origin',(11.25,11.3156378831472,-18.5));
#16817=CARTESIAN_POINT('',(8.5,11.3156378831472,-28.5));
#16818=CARTESIAN_POINT('',(8.5,11.3156378831472,-28.5));
#16819=CARTESIAN_POINT('',(9.12867965644036,9.56563788314719,-28.5));
#16820=CARTESIAN_POINT('Origin',(11.25,11.3156378831472,-28.5));
#16821=CARTESIAN_POINT('',(9.12867965644036,9.56563788314719,-20.5));
#16822=CARTESIAN_POINT('',(9.12867965644036,9.56563788314719,-28.5));
#16823=CARTESIAN_POINT('',(13.3713203435596,9.56563788314719,-20.5));
#16824=CARTESIAN_POINT('Origin',(11.25,11.3156378831472,-20.5));
#16825=CARTESIAN_POINT('',(13.3713203435596,9.56563788314719,-28.5));
#16826=CARTESIAN_POINT('',(13.3713203435596,9.56563788314719,-28.5));
#16827=CARTESIAN_POINT('',(13.3713203435596,13.0656378831472,-28.5));
#16828=CARTESIAN_POINT('Origin',(11.25,11.3156378831472,-28.5));
#16829=CARTESIAN_POINT('',(13.3713203435596,13.0656378831472,-20.5));
#16830=CARTESIAN_POINT('',(13.3713203435596,13.0656378831472,-28.5));
#16831=CARTESIAN_POINT('',(9.12867965644036,13.0656378831472,-20.5));
#16832=CARTESIAN_POINT('Origin',(11.25,11.3156378831472,-20.5));
#16833=CARTESIAN_POINT('',(9.12867965644036,13.0656378831472,-28.5));
#16834=CARTESIAN_POINT('',(9.12867965644036,13.0656378831472,-28.5));
#16835=CARTESIAN_POINT('Origin',(11.25,11.3156378831472,-28.5));
#16836=CARTESIAN_POINT('Origin',(60.5,11.2499999999998,-9.0000000000003));
#16837=CARTESIAN_POINT('',(60.5,18.236594306241,-1.5));
#16838=CARTESIAN_POINT('',(60.5,17.6580028089882,-17.0000000000006));
#16839=CARTESIAN_POINT('Origin',(60.5,11.2499999999998,-9.0000000000003));
#16840=CARTESIAN_POINT('',(62.,17.6188696014285,-3.));
#16841=CARTESIAN_POINT('Ctrl Pts',(60.5,18.2365943062411,-1.5));
#16842=CARTESIAN_POINT('Ctrl Pts',(60.6825097737065,18.2365943062411,-1.5));
#16843=CARTESIAN_POINT('Ctrl Pts',(60.8626262952116,18.2235187999567,-1.5333052678753));
#16844=CARTESIAN_POINT('Ctrl Pts',(61.2066214067746,18.1719078689624,-1.66370550137199));
#16845=CARTESIAN_POINT('Ctrl Pts',(61.3654081421642,18.1331565114149,-1.76128416762843));
#16846=CARTESIAN_POINT('Ctrl Pts',(61.6474355482113,18.0314004414372,-2.01416097458981));
#16847=CARTESIAN_POINT('Ctrl Pts',(61.7642104747049,17.9678801157231,-2.17047440300412));
#16848=CARTESIAN_POINT('Ctrl Pts',(61.8976884723899,17.8548001066011,-2.44379950745487));
#16849=CARTESIAN_POINT('Ctrl Pts',(61.9354353141332,17.8102641486262,-2.55046487110271));
#16850=CARTESIAN_POINT('Ctrl Pts',(61.9865427819248,17.7176723731834,-2.76979605527032));
#16851=CARTESIAN_POINT('Ctrl Pts',(61.999575711242,17.6697427007191,-2.88213719062229));
#16852=CARTESIAN_POINT('Ctrl Pts',(61.999996602987,17.6204611304348,-2.99631374883044));
#16853=CARTESIAN_POINT('Ctrl Pts',(62.,17.6196654289333,-2.99815690123519));
#16854=CARTESIAN_POINT('Ctrl Pts',(62.,17.6188696014285,-3.));
#16855=CARTESIAN_POINT('',(62.,17.10768725693,-15.5000000000006));
#16856=CARTESIAN_POINT('Origin',(62.,11.2499999999998,-9.0000000000003));
#16857=CARTESIAN_POINT('Ctrl Pts',(60.5,17.6580028089882,-17.0000000000006));
#16858=CARTESIAN_POINT('Ctrl Pts',(60.6849224319866,17.6580028089882,-17.0000000000006));
#16859=CARTESIAN_POINT('Ctrl Pts',(60.8675370698961,17.6460282159484,-16.9658078455989));
#16860=CARTESIAN_POINT('Ctrl Pts',(61.2149045564291,17.5988242934699,-16.8321104937404));
#16861=CARTESIAN_POINT('Ctrl Pts',(61.3748310905333,17.563515359271,-16.732437992471));
#16862=CARTESIAN_POINT('Ctrl Pts',(61.6563081266554,17.4712622036046,-16.4754110401718));
#16863=CARTESIAN_POINT('Ctrl Pts',(61.772057271832,17.4141013272841,-16.317682393564));
#16864=CARTESIAN_POINT('Ctrl Pts',(61.9020528190627,17.3133591165629,-16.0445469649045));
#16865=CARTESIAN_POINT('Ctrl Pts',(61.9381950183413,17.2744715583663,-15.9400312132836));
#16866=CARTESIAN_POINT('Ctrl Pts',(61.9870959225303,17.1937377924364,-15.7253060054237));
#16867=CARTESIAN_POINT('Ctrl Pts',(61.9995824894263,17.1520226081444,-15.6154644316008));
#16868=CARTESIAN_POINT('Ctrl Pts',(61.9999965682669,17.1091102687603,-15.5037050301089));
#16869=CARTESIAN_POINT('Ctrl Pts',(62.,17.1083988194954,-15.5018524937658));
#16870=CARTESIAN_POINT('Ctrl Pts',(62.,17.10768725693,-15.5000000000006));
#16871=CARTESIAN_POINT('Origin',(62.,11.2500000000003,-9.00000000000028));
#16872=CARTESIAN_POINT('',(60.5,4.84199719101188,-17.0000000000006));
#16873=CARTESIAN_POINT('',(60.5,4.26340569375895,-1.5));
#16874=CARTESIAN_POINT('Origin',(60.5,11.2500000000003,-9.00000000000028));
#16875=CARTESIAN_POINT('',(48.,4.26340569375895,-1.5));
#16876=CARTESIAN_POINT('',(62.,4.26340569375895,-1.5));
#16877=CARTESIAN_POINT('',(48.,4.84199719101187,-17.0000000000006));
#16878=CARTESIAN_POINT('Origin',(48.,11.2500000000003,-9.00000000000028));
#16879=CARTESIAN_POINT('',(62.,4.84199719101188,-17.0000000000006));
#16880=CARTESIAN_POINT('Origin',(48.,11.25,-9.25));
#16881=CARTESIAN_POINT('',(48.,3.88029851350817,-0.75));
#16882=CARTESIAN_POINT('',(48.,4.84687576256716,-18.5));
#16883=CARTESIAN_POINT('Origin',(48.,11.25,-9.25));
#16884=CARTESIAN_POINT('',(37.,3.88029851350817,-0.75));
#16885=CARTESIAN_POINT('',(48.,3.88029851350817,-0.75));
#16886=CARTESIAN_POINT('',(37.,0.,-9.25));
#16887=CARTESIAN_POINT('Origin',(37.,11.25,-9.25));
#16888=CARTESIAN_POINT('',(37.,4.84687576256715,-18.5));
#16889=CARTESIAN_POINT('Origin',(37.,11.25,-9.25));
#16890=CARTESIAN_POINT('',(48.,4.84687576256716,-18.5));
#16891=CARTESIAN_POINT('Origin',(11.25,11.3156378831472,10.));
#16892=CARTESIAN_POINT('',(14.,11.3156378831472,0.));
#16893=CARTESIAN_POINT('Origin',(11.25,11.3156378831472,0.));
#16894=CARTESIAN_POINT('',(14.,11.3156378831472,10.));
#16895=CARTESIAN_POINT('',(14.,11.3156378831472,10.));
#16896=CARTESIAN_POINT('',(13.3713203435596,9.56563788314719,10.));
#16897=CARTESIAN_POINT('Origin',(11.25,11.3156378831472,10.));
#16898=CARTESIAN_POINT('',(13.3713203435596,9.56563788314719,2.));
#16899=CARTESIAN_POINT('',(13.3713203435596,9.56563788314719,10.));
#16900=CARTESIAN_POINT('',(9.12867965644036,9.56563788314719,2.));
#16901=CARTESIAN_POINT('Origin',(11.25,11.3156378831472,2.));
#16902=CARTESIAN_POINT('',(9.12867965644036,9.56563788314719,10.));
#16903=CARTESIAN_POINT('',(9.12867965644036,9.56563788314719,10.));
#16904=CARTESIAN_POINT('',(9.12867965644036,13.0656378831472,10.));
#16905=CARTESIAN_POINT('Origin',(11.25,11.3156378831472,10.));
#16906=CARTESIAN_POINT('',(9.12867965644036,13.0656378831472,2.));
#16907=CARTESIAN_POINT('',(9.12867965644036,13.0656378831472,10.));
#16908=CARTESIAN_POINT('',(13.3713203435596,13.0656378831472,2.));
#16909=CARTESIAN_POINT('Origin',(11.25,11.3156378831472,2.));
#16910=CARTESIAN_POINT('',(13.3713203435596,13.0656378831472,10.));
#16911=CARTESIAN_POINT('',(13.3713203435596,13.0656378831472,10.));
#16912=CARTESIAN_POINT('Origin',(11.25,11.3156378831472,10.));
#16913=CARTESIAN_POINT('Origin',(3.,19.5,-18.5));
#16914=CARTESIAN_POINT('',(37.,0.,-18.5));
#16915=CARTESIAN_POINT('',(37.,0.,-18.5));
#16916=CARTESIAN_POINT('',(3.,0.,-18.5));
#16917=CARTESIAN_POINT('',(3.,0.,-18.5));
#16918=CARTESIAN_POINT('',(0.,3.,-18.5));
#16919=CARTESIAN_POINT('Origin',(3.,3.,-18.5));
#16920=CARTESIAN_POINT('',(4.33680868994202E-16,19.5,-18.5));
#16921=CARTESIAN_POINT('',(0.,3.,-18.5));
#16922=CARTESIAN_POINT('',(3.,22.5,-18.5));
#16923=CARTESIAN_POINT('Origin',(3.,19.5,-18.5));
#16924=CARTESIAN_POINT('',(37.,22.5,-18.5));
#16925=CARTESIAN_POINT('',(3.,22.5,-18.5));
#16926=CARTESIAN_POINT('',(37.,17.6531242374329,-18.5));
#16927=CARTESIAN_POINT('',(37.,0.,-18.5));
#16928=CARTESIAN_POINT('',(48.,17.6531242374329,-18.5));
#16929=CARTESIAN_POINT('',(48.,17.6531242374329,-18.5));
#16930=CARTESIAN_POINT('',(48.,3.39234813079909E-15,-18.5));
#16931=CARTESIAN_POINT('Origin',(0.,3.,-18.5));
#16932=CARTESIAN_POINT('',(4.33680868994202E-16,19.5,0.));
#16933=CARTESIAN_POINT('',(0.,3.,0.));
#16934=CARTESIAN_POINT('',(0.,3.,0.));
#16935=CARTESIAN_POINT('',(4.33680868994202E-16,19.5,-18.5));
#16936=CARTESIAN_POINT('',(0.,3.,-18.5));
#16937=CARTESIAN_POINT('',(0.,9.,-10.75));
#16938=CARTESIAN_POINT('',(0.,9.,-7.75));
#16939=CARTESIAN_POINT('',(0.,9.,-10.75));
#16940=CARTESIAN_POINT('',(0.,14.,-10.75));
#16941=CARTESIAN_POINT('',(0.,14.,-10.75));
#16942=CARTESIAN_POINT('',(0.,14.,-7.75));
#16943=CARTESIAN_POINT('',(0.,14.,-10.75));
#16944=CARTESIAN_POINT('',(0.,14.,-7.75));
#16945=CARTESIAN_POINT('Origin',(11.25,11.3156378831472,10.));
#16946=CARTESIAN_POINT('',(14.4729344439275,9.56563788314719,10.));
#16947=CARTESIAN_POINT('',(14.4729344439275,13.0656378831472,10.));
#16948=CARTESIAN_POINT('Origin',(48.,11.25,-9.25));
#16949=CARTESIAN_POINT('',(48.,18.6197014864918,-0.75));
#16950=CARTESIAN_POINT('Origin',(48.,11.25,-9.25));
#16951=CARTESIAN_POINT('',(48.,-0.293389173340333,-0.75));
#16952=CARTESIAN_POINT('',(48.,18.236594306241,-1.5));
#16953=CARTESIAN_POINT('',(48.,18.236594306241,-1.5));
#16954=CARTESIAN_POINT('',(48.,17.6580028089882,-17.0000000000006));
#16955=CARTESIAN_POINT('Origin',(48.,11.2499999999998,-9.0000000000003));
#16956=CARTESIAN_POINT('',(48.,4.84199719101188,-17.0000000000006));
#16957=CARTESIAN_POINT('Origin',(48.,11.25,-9.25));
#16958=CARTESIAN_POINT('',(37.,22.5,-9.25));
#16959=CARTESIAN_POINT('Origin',(37.,11.25,-9.25));
#16960=CARTESIAN_POINT('',(37.,18.6197014864918,-0.75));
#16961=CARTESIAN_POINT('Origin',(37.,11.25,-9.25));
#16962=CARTESIAN_POINT('',(48.,18.6197014864918,-0.75));
#16963=CARTESIAN_POINT('Origin',(37.,0.,-18.5));
#16964=CARTESIAN_POINT('',(37.,0.,-18.5));
#16965=CARTESIAN_POINT('Origin',(37.,0.,-18.5));
#16966=CARTESIAN_POINT('',(37.,22.5,0.));
#16967=CARTESIAN_POINT('',(37.,22.5,-18.5));
#16968=CARTESIAN_POINT('',(37.,0.,0.));
#16969=CARTESIAN_POINT('',(37.,0.,0.));
#16970=CARTESIAN_POINT('',(37.,0.,-18.5));
#16971=CARTESIAN_POINT('',(37.,-0.293389173340335,-0.75));
#16972=CARTESIAN_POINT('Origin',(37.,0.,-18.5));
#16973=CARTESIAN_POINT('',(37.,22.5,-18.5));
#16974=CARTESIAN_POINT('Origin',(3.,0.,-18.5));
#16975=CARTESIAN_POINT('',(3.,0.,0.));
#16976=CARTESIAN_POINT('',(3.,0.,0.));
#16977=CARTESIAN_POINT('',(3.,0.,-18.5));
#16978=CARTESIAN_POINT('Origin',(3.,3.,-18.5));
#16979=CARTESIAN_POINT('Origin',(3.,3.,0.));
#16980=CARTESIAN_POINT('Origin',(3.,19.5,-18.5));
#16981=CARTESIAN_POINT('',(3.,22.5,0.));
#16982=CARTESIAN_POINT('Origin',(3.,19.5,0.));
#16983=CARTESIAN_POINT('',(3.,22.5,-18.5));
#16984=CARTESIAN_POINT('Origin',(3.,22.5,-18.5));
#16985=CARTESIAN_POINT('',(3.,22.5,0.));
#16986=CARTESIAN_POINT('Origin',(3.,19.5,0.));
#16987=CARTESIAN_POINT('Origin',(37.,-0.293389173340335,-0.75));
#16988=CARTESIAN_POINT('Origin',(62.,11.2499999999998,-9.0000000000003));
#16989=CARTESIAN_POINT('',(62.,18.236594306241,-1.5));
#16990=CARTESIAN_POINT('',(62.,17.6580028089882,-17.0000000000006));
#16991=CARTESIAN_POINT('Origin',(62.,18.236594306241,-1.5));
#16992=CARTESIAN_POINT('',(60.5,18.236594306241,-1.5));
#16993=CARTESIAN_POINT('Origin',(62.,4.84199719101188,-17.0000000000006));
#16994=CARTESIAN_POINT('',(60.5,4.84199719101188,-17.0000000000006));
#16995=CARTESIAN_POINT('Origin',(62.,11.2499999999998,-9.0000000000003));
#16996=CARTESIAN_POINT('',(62.,4.88113039857151,-3.));
#16997=CARTESIAN_POINT('',(62.,5.39231274307003,-15.5000000000006));
#16998=CARTESIAN_POINT('Origin',(62.,11.2500000000003,-9.00000000000028));
#16999=CARTESIAN_POINT('',(62.,17.6580028089882,-15.5000000000006));
#17000=CARTESIAN_POINT('',(62.,4.26340569375895,-3.));
#17001=CARTESIAN_POINT('Origin',(60.5,11.2499999999998,-3.));
#17002=CARTESIAN_POINT('Ctrl Pts',(62.,4.8811303985715,-3.));
#17003=CARTESIAN_POINT('Ctrl Pts',(62.,4.88033457106672,-2.99815690123521));
#17004=CARTESIAN_POINT('Ctrl Pts',(61.999996602987,4.87953886956515,-2.99631374883042));
#17005=CARTESIAN_POINT('Ctrl Pts',(61.999575711242,4.8302572992812,-2.88213719062315));
#17006=CARTESIAN_POINT('Ctrl Pts',(61.9865427819249,4.78232762681674,-2.76979605527046));
#17007=CARTESIAN_POINT('Ctrl Pts',(61.9354353141332,4.68973585137378,-2.55046487110269));
#17008=CARTESIAN_POINT('Ctrl Pts',(61.8976884723899,4.64519989339895,-2.44379950745486));
#17009=CARTESIAN_POINT('Ctrl Pts',(61.7642104747049,4.53211988427689,-2.17047440300411));
#17010=CARTESIAN_POINT('Ctrl Pts',(61.6474355482113,4.46859955856276,-2.01416097458981));
#17011=CARTESIAN_POINT('Ctrl Pts',(61.3654081421642,4.3668434885851,-1.76128416762844));
#17012=CARTESIAN_POINT('Ctrl Pts',(61.2066214067746,4.32809213103761,-1.66370550137199));
#17013=CARTESIAN_POINT('Ctrl Pts',(60.8626262952117,4.27648120004334,-1.5333052678753));
#17014=CARTESIAN_POINT('Ctrl Pts',(60.6825097737065,4.26340569375894,-1.5));
#17015=CARTESIAN_POINT('Ctrl Pts',(60.5,4.26340569375894,-1.5));
#17016=CARTESIAN_POINT('Origin',(60.5,11.2500000000003,-9.00000000000028));
#17017=CARTESIAN_POINT('Ctrl Pts',(62.,5.39231274307,-15.5000000000005));
#17018=CARTESIAN_POINT('Ctrl Pts',(62.,5.39160118050427,-15.5018524937667));
#17019=CARTESIAN_POINT('Ctrl Pts',(61.9999965682669,5.39088973123915,-15.5037050301105));
#17020=CARTESIAN_POINT('Ctrl Pts',(61.9995824894261,5.34797739185418,-15.6154644316047));
#17021=CARTESIAN_POINT('Ctrl Pts',(61.9870959225299,5.30626220756289,-15.7253060054257));
#17022=CARTESIAN_POINT('Ctrl Pts',(61.938195018341,5.22552844163345,-15.9400312132845));
#17023=CARTESIAN_POINT('Ctrl Pts',(61.9020528190626,5.186640883437,-16.0445469649049));
#17024=CARTESIAN_POINT('Ctrl Pts',(61.772057271832,5.08589867271599,-16.317682393564));
#17025=CARTESIAN_POINT('Ctrl Pts',(61.6563081266553,5.02873779639548,-16.4754110401719));
#17026=CARTESIAN_POINT('Ctrl Pts',(61.3748310905333,4.93648464072909,-16.732437992471));
#17027=CARTESIAN_POINT('Ctrl Pts',(61.2149045564291,4.90117570653016,-16.8321104937404));
#17028=CARTESIAN_POINT('Ctrl Pts',(60.8675370698961,4.85397178405163,-16.9658078455989));
#17029=CARTESIAN_POINT('Ctrl Pts',(60.6849224319866,4.84199719101184,-17.0000000000006));
#17030=CARTESIAN_POINT('Ctrl Pts',(60.5,4.84199719101184,-17.0000000000006));
#17031=CARTESIAN_POINT('Origin',(60.5,11.2499999999998,-15.5000000000006));
#17032=CARTESIAN_POINT('Origin',(11.25,11.3156378831472,-28.5));
#17033=CARTESIAN_POINT('',(11.25,9.56563788314719,-28.5));
#17034=CARTESIAN_POINT('',(11.25,13.0656378831472,-28.5));
#17035=CARTESIAN_POINT('Origin',(14.4729344439275,13.0656378831472,-20.5));
#17036=CARTESIAN_POINT('',(14.4729344439275,13.0656378831472,-20.5));
#17037=CARTESIAN_POINT('Origin',(14.4729344439275,13.0656378831472,-20.5));
#17038=CARTESIAN_POINT('Origin',(14.4729344439275,7.8996035579007,-20.5));
#17039=CARTESIAN_POINT('',(14.4729344439275,9.56563788314719,-20.5));
#17040=CARTESIAN_POINT('Origin',(14.4729344439275,9.56563788314719,-20.5));
#17041=CARTESIAN_POINT('Origin',(14.4729344439275,13.0656378831472,2.));
#17042=CARTESIAN_POINT('',(14.4729344439275,13.0656378831472,2.));
#17043=CARTESIAN_POINT('Origin',(14.4729344439275,13.0656378831472,2.));
#17044=CARTESIAN_POINT('Origin',(14.4729344439275,9.56563788314719,2.));
#17045=CARTESIAN_POINT('',(14.4729344439275,9.56563788314719,2.));
#17046=CARTESIAN_POINT('Origin',(14.4729344439275,7.8996035579007,2.));
#17047=CARTESIAN_POINT('Origin',(-4.5,14.,-10.75));
#17048=CARTESIAN_POINT('',(-4.5,9.,-10.75));
#17049=CARTESIAN_POINT('',(-4.5,9.,-10.75));
#17050=CARTESIAN_POINT('',(-4.5,14.,-10.75));
#17051=CARTESIAN_POINT('',(-4.5,14.,-10.75));
#17052=CARTESIAN_POINT('',(-4.5,14.,-10.75));
#17053=CARTESIAN_POINT('Origin',(-4.5,9.,-10.75));
#17054=CARTESIAN_POINT('',(-4.5,9.,-7.75));
#17055=CARTESIAN_POINT('',(-4.5,9.,-7.75));
#17056=CARTESIAN_POINT('',(-4.5,9.,-10.75));
#17057=CARTESIAN_POINT('Origin',(-4.5,14.,-7.75));
#17058=CARTESIAN_POINT('',(-4.5,14.,-7.75));
#17059=CARTESIAN_POINT('',(-4.5,14.,-7.75));
#17060=CARTESIAN_POINT('',(-4.5,14.,-7.75));
#17061=CARTESIAN_POINT('Origin',(-4.5,14.,-10.75));
#17062=CARTESIAN_POINT('',(-4.5,14.,-10.75));
#17063=CARTESIAN_POINT('Origin',(-4.5,9.,-10.75));
#17064=CARTESIAN_POINT('Origin',(22.,11.3156378831472,-20.5));
#18840=UNCERTAINTY_MEASURE_WITH_UNIT(LENGTH_MEASURE(0.01),#18868,
'DISTANCE_ACCURACY_VALUE',
'Maximum model space distance between geometric entities at asserted c
onnectivities');
#18849=UNCERTAINTY_MEASURE_WITH_UNIT(LENGTH_MEASURE(0.01),#18868,
'DISTANCE_ACCURACY_VALUE',
'Maximum model space distance between geometric entities at asserted c
onnectivities');
#18858=(
GEOMETRIC_REPRESENTATION_CONTEXT(3)
GLOBAL_UNCERTAINTY_ASSIGNED_CONTEXT((#18840))
GLOBAL_UNIT_ASSIGNED_CONTEXT((#18868,#18870,#18871))
REPRESENTATION_CONTEXT('','3D')
);
#18867=(
GEOMETRIC_REPRESENTATION_CONTEXT(3)
GLOBAL_UNCERTAINTY_ASSIGNED_CONTEXT((#18849))
GLOBAL_UNIT_ASSIGNED_CONTEXT((#18868,#18870,#18871))
REPRESENTATION_CONTEXT('','3D')
);
#18868=(
LENGTH_UNIT()
NAMED_UNIT(*)
SI_UNIT(.MILLI.,.METRE.)
);
#18870=(
NAMED_UNIT(*)
PLANE_ANGLE_UNIT()
SI_UNIT($,.RADIAN.)
);
#18871=(
NAMED_UNIT(*)
SI_UNIT($,.STERADIAN.)
SOLID_ANGLE_UNIT()
);
#18880=SHAPE_DEFINITION_REPRESENTATION(#18897,#18942);
#18897=PRODUCT_DEFINITION_SHAPE('',$,#18960);
#18942=SHAPE_REPRESENTATION('',(#11578),#18858);
#18951=PRODUCT_DEFINITION_CONTEXT('part definition',#19004,'design');
#18960=PRODUCT_DEFINITION('motor','Motor',#18977,#18951);
#18977=PRODUCT_DEFINITION_FORMATION('',$,#19014);
#19004=APPLICATION_CONTEXT(
'Core Data for Automotive Mechanical Design Process');
#19005=PRODUCT_CONTEXT('part definition',#19004,'mechanical');
#19014=PRODUCT('motor','Motor',$,(#19005));
#19026=PRESENTATION_STYLE_ASSIGNMENT((#19032));
#19032=SURFACE_STYLE_USAGE(.BOTH.,#19038);
#19038=SURFACE_SIDE_STYLE('',(#19044));
#19044=SURFACE_STYLE_FILL_AREA(#19050);
#19050=FILL_AREA_STYLE('Opaque(227,224,212)',(#19056));
#19056=FILL_AREA_STYLE_COLOUR('Opaque(227,224,212)',#19062);
#19062=COLOUR_RGB('Opaque(227,224,212)',0.890196078431372,0.87843137254902,
0.831372549019608);
ENDSEC;
END-ISO-10303-21;
